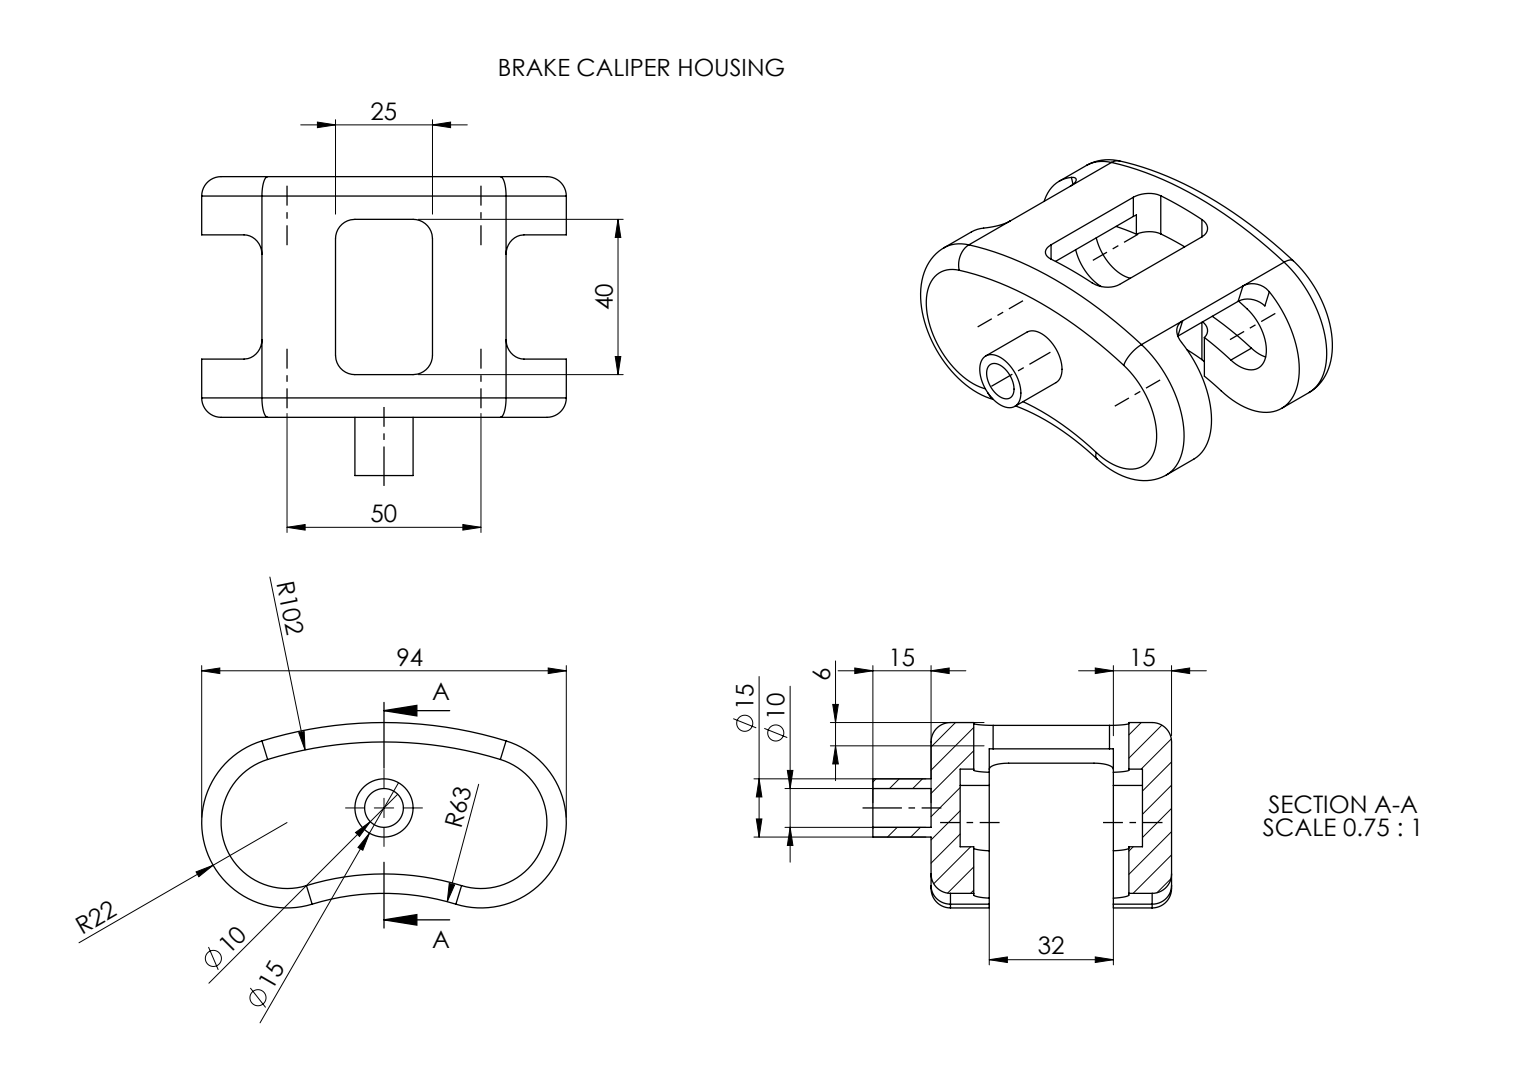
ISO-10303-21;
HEADER;
FILE_DESCRIPTION (('STEP AP214'),
    '1' );
FILE_NAME ('brake caliper housing.step',
    '2026-10-02T06:35:35',
    ( '' ),
    ( '' ),
    'SwSTEP 2.0',
    'SolidWorks 2026',
    '' );
FILE_SCHEMA (( 'AUTOMOTIVE_DESIGN' ));
ENDSEC;

DATA;
#2=DIRECTION ( 'NONE',  ( -1.000000000000000000, 0.000000000000000000, 0.000000000000000000 ) ) ;
#5=DIRECTION ( 'NONE',  ( -1.000000000000000000, 0.000000000000000000, 0.000000000000000000 ) ) ;
#22=AXIS2_PLACEMENT_3D ( 'NONE', #10002, #1881, #9007 ) ;
#27=VERTEX_POINT ( 'NONE', #8027 ) ;
#36=DIRECTION ( 'NONE',  ( -0.000000000000000000, -0.000000000000000000, -1.000000000000000000 ) ) ;
#37=CYLINDRICAL_SURFACE ( 'NONE', #355, 22.00000000000001421 ) ;
#47=CARTESIAN_POINT ( 'NONE',  ( 47.00000000000001421, 81.24038404635960831, -31.00000000000000000 ) ) ;
#48=FACE_BOUND ( 'NONE', #7708, .T. ) ;
#52=CARTESIAN_POINT ( 'NONE',  ( 36.08010649850015739, 100.2464683348682541, -16.00000000000000000 ) ) ;
#63=AXIS2_PLACEMENT_3D ( 'NONE', #8204, #12550, #5924 ) ;
#69=ADVANCED_FACE ( 'NONE', ( #14874 ), #12670, .F. ) ;
#73=EDGE_CURVE ( 'NONE', #4839, #9064, #14954, .T. ) ;
#82=CIRCLE ( 'NONE', #4216, 63.00000000000000000 ) ;
#86=LINE ( 'NONE', #9270, #8545 ) ;
#88=FACE_OUTER_BOUND ( 'NONE', #3167, .T. ) ;
#92=CARTESIAN_POINT ( 'NONE',  ( -10.00610186947451474, 106.5314655734664910, -19.33904518629106306 ) ) ;
#94=B_SPLINE_CURVE_WITH_KNOTS ( 'NONE', 3,
 ( #9442, #2468, #4910, #4826, #14091, #9801, #11106, #8665, #3618, #8738, #13380, #3696, #12955, #2552, #2981, #7235, #10661, #9522, #3776, #4761 ),
 .UNSPECIFIED., .F., .F.,
 ( 4, 2, 2, 2, 2, 2, 2, 2, 2, 4 ),
 ( 0.000000000000000000, 0.0009783709435495714819, 0.001467556415324351151, 0.001956741887099130821, 0.002935112830648695798, 0.003913483774198260774, 0.004891854717747825751, 0.005870225661297390728, 0.006848596604846954837, 0.007826967548396519814 ),
 .UNSPECIFIED. ) ;
#97=ORIENTED_EDGE ( 'NONE', *, *, #2089, .T. ) ;
#99=AXIS2_PLACEMENT_3D ( 'NONE', #4932, #13204, #7338 ) ;
#105=PLANE ( 'NONE',  #6564 ) ;
#111=DIRECTION ( 'NONE',  ( 1.000000000000000000, 0.000000000000000000, 0.000000000000000000 ) ) ;
#122=FACE_OUTER_BOUND ( 'NONE', #11782, .T. ) ;
#127=CARTESIAN_POINT ( 'NONE',  ( -10.20439220990035345, 94.45068983291282905, 19.21516791372541633 ) ) ;
#135=CARTESIAN_POINT ( 'NONE',  ( 12.50000000000000000, 40.62019202317980415, -16.00000000000000000 ) ) ;
#137=CARTESIAN_POINT ( 'NONE',  ( 10.21169758550232309, 62.16852661215632025, 19.23993411931846254 ) ) ;
#138=ORIENTED_EDGE ( 'NONE', *, *, #8514, .T. ) ;
#143=VERTEX_POINT ( 'NONE', #12163 ) ;
#155=ADVANCED_FACE ( 'NONE', ( #11017 ), #623, .F. ) ;
#179=CARTESIAN_POINT ( 'NONE',  ( 35.00000000000000000, 81.24038404635960831, 16.00000000000000000 ) ) ;
#200=DIRECTION ( 'NONE',  ( 0.000000000000000000, 0.000000000000000000, -1.000000000000000000 ) ) ;
#201=CARTESIAN_POINT ( 'NONE',  ( 11.10302805179279240, 62.01554028455485224, 18.51404809149990882 ) ) ;
#205=ORIENTED_EDGE ( 'NONE', *, *, #9389, .F. ) ;
#216=DIRECTION ( 'NONE',  ( 0.000000000000000000, 1.000000000000000000, 0.000000000000000000 ) ) ;
#220=ADVANCED_FACE ( 'NONE', ( #7246 ), #8324, .F. ) ;
#223=CARTESIAN_POINT ( 'NONE',  ( 25.00000000000000000, 81.24038404635960831, 26.00000000000000000 ) ) ;
#230=CARTESIAN_POINT ( 'NONE',  ( 12.39897948556635754, 61.76783392443436327, 16.00000000000000000 ) ) ;
#245=EDGE_LOOP ( 'NONE', ( #12911, #1425, #6697, #4365 ) ) ;
#253=FACE_OUTER_BOUND ( 'NONE', #11246, .T. ) ;
#257=AXIS2_PLACEMENT_3D ( 'NONE', #4931, #14259, #10909 ) ;
#259=VERTEX_POINT ( 'NONE', #10384 ) ;
#261=VECTOR ( 'NONE', #10408, 1000.000000000000000 ) ;
#266=EDGE_CURVE ( 'NONE', #4701, #13246, #688, .T. ) ;
#273=EDGE_CURVE ( 'NONE', #3532, #8404, #4570, .T. ) ;
#293=DIRECTION ( 'NONE',  ( 0.000000000000000000, 0.000000000000000000, -1.000000000000000000 ) ) ;
#296=CARTESIAN_POINT ( 'NONE',  ( 0.000000000000000000, 0.000000000000000000, 0.000000000000000000 ) ) ;
#298=FACE_OUTER_BOUND ( 'NONE', #14007, .T. ) ;
#304=AXIS2_PLACEMENT_3D ( 'NONE', #341, #1635, #4982 ) ;
#308=DIRECTION ( 'NONE',  ( 1.000000000000000000, 0.000000000000000000, 0.000000000000000000 ) ) ;
#310=CARTESIAN_POINT ( 'NONE',  ( 34.93100731845030538, 100.8740421756369585, -15.84356320956305986 ) ) ;
#315=AXIS2_PLACEMENT_3D ( 'NONE', #10797, #13156, #2521 ) ;
#320=ADVANCED_FACE ( 'NONE', ( #5891 ), #10531, .F. ) ;
#323=CARTESIAN_POINT ( 'NONE',  ( -9.716053034936795285, 106.5583837859906424, -19.49385781195229228 ) ) ;
#326=CARTESIAN_POINT ( 'NONE',  ( 31.47058823529413374, 102.2673069760056563, -31.00000000000000000 ) ) ;
#330=DIRECTION ( 'NONE',  ( 0.000000000000000000, 0.000000000000000000, -1.000000000000000000 ) ) ;
#331=VERTEX_POINT ( 'NONE', #8544 ) ;
#335=CARTESIAN_POINT ( 'NONE',  ( -33.08820577230232374, 101.7009610928537171, -14.78158739605038186 ) ) ;
#337=VERTEX_POINT ( 'NONE', #667 ) ;
#341=CARTESIAN_POINT ( 'NONE',  ( 25.00000000000000000, 81.24038404635960831, -31.00000000000000000 ) ) ;
#342=CIRCLE ( 'NONE', #8819, 75.00000000000001421 ) ;
#350=CARTESIAN_POINT ( 'NONE',  ( 10.43254889841015753, 62.13061131512487378, -19.05984907584257115 ) ) ;
#355=AXIS2_PLACEMENT_3D ( 'NONE', #4755, #11596, #10653 ) ;
#366=ORIENTED_EDGE ( 'NONE', *, *, #266, .F. ) ;
#369=AXIS2_PLACEMENT_3D ( 'NONE', #5329, #6524, #6684 ) ;
#370=ORIENTED_EDGE ( 'NONE', *, *, #5461, .F. ) ;
#373=DIRECTION ( 'NONE',  ( 0.000000000000000000, 0.000000000000000000, -1.000000000000000000 ) ) ;
#376=DIRECTION ( 'NONE',  ( 0.000000000000000000, 0.000000000000000000, 1.000000000000000000 ) ) ;
#377=DIRECTION ( 'NONE',  ( 1.000000000000000000, 0.000000000000000000, 0.000000000000000000 ) ) ;
#379=DIRECTION ( 'NONE',  ( -0.000000000000000000, -0.000000000000000000, -1.000000000000000000 ) ) ;
#382=EDGE_CURVE ( 'NONE', #697, #1597, #12234, .T. ) ;
#383=ORIENTED_EDGE ( 'NONE', *, *, #10951, .T. ) ;
#394=AXIS2_PLACEMENT_3D ( 'NONE', #10510, #36, #111 ) ;
#397=CARTESIAN_POINT ( 'NONE',  ( -11.83867104060235853, 106.3432143034623749, -17.50653253748098948 ) ) ;
#405=CARTESIAN_POINT ( 'NONE',  ( 12.46631608856921325, 100.2277185551817951, 15.67011936326128563 ) ) ;
#411=CARTESIAN_POINT ( 'NONE',  ( -31.71893208106490292, 102.1896529572239700, -12.62523369519216310 ) ) ;
#412=DIRECTION ( 'NONE',  ( 1.000000000000000000, 0.000000000000000000, 0.000000000000000000 ) ) ;
#428=CARTESIAN_POINT ( 'NONE',  ( -29.82779671029264890, 96.49509599019863515, -12.13403317654896973 ) ) ;
#450=CARTESIAN_POINT ( 'NONE',  ( -33.23060097332287199, 95.37689352056797532, 15.83317473434553690 ) ) ;
#453=LINE ( 'NONE', #9482, #11663 ) ;
#465=ORIENTED_EDGE ( 'NONE', *, *, #515, .F. ) ;
#467=B_SPLINE_CURVE_WITH_KNOTS ( 'NONE', 3,
 ( #4608, #10222, #15012, #14864, #7939, #12736, #1129, #12580, #13880, #3468, #13799, #2170, #3388, #6787, #11451, #12658, #1049, #8088 ),
 .UNSPECIFIED., .F., .F.,
 ( 4, 2, 2, 2, 2, 2, 2, 2, 4 ),
 ( 0.001002962753164633562, 0.001858089309406475969, 0.002713215865648318376, 0.003568342421890161216, 0.004423468978132004056, 0.005278595534373846029, 0.006133722090615688870, 0.006988848646857530843, 0.007843975203099373683 ),
 .UNSPECIFIED. ) ;
#470=CARTESIAN_POINT ( 'NONE',  ( 12.50000000000000000, 100.2235002382176248, 15.00000000000000000 ) ) ;
#478=DIRECTION ( 'NONE',  ( 0.000000000000000000, 0.000000000000000000, 1.000000000000000000 ) ) ;
#495=CARTESIAN_POINT ( 'NONE',  ( 11.45661564179884451, 61.94983405580222069, -18.07016506142804246 ) ) ;
#500=ORIENTED_EDGE ( 'NONE', *, *, #5316, .T. ) ;
#506=EDGE_CURVE ( 'NONE', #259, #13406, #11535, .T. ) ;
#508=VERTEX_POINT ( 'NONE', #11134 ) ;
#514=ORIENTED_EDGE ( 'NONE', *, *, #273, .T. ) ;
#515=EDGE_CURVE ( 'NONE', #15011, #5203, #11902, .T. ) ;
#527=EDGE_LOOP ( 'NONE', ( #759, #3459, #4325, #3794, #1827, #1753, #97, #3731 ) ) ;
#529=( GEOMETRIC_REPRESENTATION_CONTEXT ( 3 ) GLOBAL_UNCERTAINTY_ASSIGNED_CONTEXT ( ( #3045 ) ) GLOBAL_UNIT_ASSIGNED_CONTEXT ( ( #9128, #5633, #14911 ) ) REPRESENTATION_CONTEXT ( 'NONE', 'WORKASPACE' ) );
#530=EDGE_CURVE ( 'NONE', #7196, #1593, #12249, .T. ) ;
#531=CARTESIAN_POINT ( 'NONE',  ( 33.08545438203831424, 101.7020459634810976, -14.77901645503695605 ) ) ;
#532=EDGE_CURVE ( 'NONE', #4198, #5509, #6823, .T. ) ;
#564=LINE ( 'NONE', #14460, #13714 ) ;
#575=DIRECTION ( 'NONE',  ( 1.000000000000000000, 0.000000000000000000, 0.000000000000000000 ) ) ;
#576=PLANE ( 'NONE',  #9518 ) ;
#578=CARTESIAN_POINT ( 'NONE',  ( -30.00974697327757212, 96.43868009418278575, -12.76250177908513983 ) ) ;
#597=ADVANCED_FACE ( 'NONE', ( #8308 ), #37, .T. ) ;
#599=LINE ( 'NONE', #5072, #14330 ) ;
#609=ORIENTED_EDGE ( 'NONE', *, *, #9991, .T. ) ;
#613=CARTESIAN_POINT ( 'NONE',  ( -31.56843276583338209, 95.94012674102927463, 14.97885581718526105 ) ) ;
#623=CYLINDRICAL_SURFACE ( 'NONE', #7215, 4.999999999999998224 ) ;
#627=VECTOR ( 'NONE', #12367, 1000.000000000000000 ) ;
#629=CARTESIAN_POINT ( 'NONE',  ( 32.78625152019765210, 95.53054288192240051, -15.68243957109766207 ) ) ;
#638=AXIS2_PLACEMENT_3D ( 'NONE', #14300, #5118, #7308 ) ;
#641=CARTESIAN_POINT ( 'NONE',  ( -12.39897948556635754, 94.18739463280904545, 16.00000000000000000 ) ) ;
#643=EDGE_LOOP ( 'NONE', ( #12832, #6192, #9404, #8598 ) ) ;
#646=CARTESIAN_POINT ( 'NONE',  ( 25.00000000000000000, 81.24038404635960831, 31.00000000000000000 ) ) ;
#650=ORIENTED_EDGE ( 'NONE', *, *, #11602, .F. ) ;
#658=CARTESIAN_POINT ( 'NONE',  ( 8.076099607191862262, 62.48290387921808531, -20.00000000000000355 ) ) ;
#659=CARTESIAN_POINT ( 'NONE',  ( 30.00000000000000355, 97.48846085563152997, 31.00000000000000000 ) ) ;
#666=CARTESIAN_POINT ( 'NONE',  ( -7.499999999999996447, 85.00000000000000000, 31.00000000000000000 ) ) ;
#667=CARTESIAN_POINT ( 'NONE',  ( 29.70588235294119173, 96.53269163155674448, 10.99999999999999645 ) ) ;
#672=CARTESIAN_POINT ( 'NONE',  ( -12.46631608856921325, 100.2277185551817951, -15.67011936326128563 ) ) ;
#673=CARTESIAN_POINT ( 'NONE',  ( -19.99999999999998934, 64.99230723708770086, 31.00000000000000000 ) ) ;
#674=APPLICATION_CONTEXT ( 'automotive_design' ) ;
#675=( LENGTH_UNIT ( ) NAMED_UNIT ( * ) SI_UNIT ( .MILLI., .METRE. ) );
#681=AXIS2_PLACEMENT_3D ( 'NONE', #14508, #12588, #11545 ) ;
#684=CARTESIAN_POINT ( 'NONE',  ( -33.83210567914650113, 95.16559600367024530, 15.96768719852781615 ) ) ;
#686=EDGE_CURVE ( 'NONE', #1445, #27, #6861, .T. ) ;
#687=DIRECTION ( 'NONE',  ( -0.000000000000000000, -0.000000000000000000, -1.000000000000000000 ) ) ;
#688=CIRCLE ( 'NONE', #3352, 75.00000000000001421 ) ;
#697=VERTEX_POINT ( 'NONE', #5872 ) ;
#698=CARTESIAN_POINT ( 'NONE',  ( 0.000000000000000000, 0.000000000000000000, 31.00000000000000000 ) ) ;
#699=EDGE_CURVE ( 'NONE', #5509, #721, #10511, .T. ) ;
#705=CARTESIAN_POINT ( 'NONE',  ( -11.47921512510733422, 94.30438942219511489, -18.08174836683881992 ) ) ;
#714=DIRECTION ( 'NONE',  ( 0.000000000000000000, 0.000000000000000000, 1.000000000000000000 ) ) ;
#717=DIRECTION ( 'NONE',  ( -0.000000000000000000, -0.000000000000000000, 1.000000000000000000 ) ) ;
#720=ADVANCED_FACE ( 'NONE', ( #6388 ), #10963, .T. ) ;
#721=VERTEX_POINT ( 'NONE', #13248 ) ;
#725=CARTESIAN_POINT ( 'NONE',  ( 11.83526203526748333, 106.3435961965382290, -17.51264358390114140 ) ) ;
#730=ORIENTED_EDGE ( 'NONE', *, *, #3331, .F. ) ;
#736=CARTESIAN_POINT ( 'NONE',  ( 35.50766591049263354, 100.5715065882092460, 15.96896126722778497 ) ) ;
#739=EDGE_LOOP ( 'NONE', ( #11744, #3948, #14361, #10298 ) ) ;
#754=CARTESIAN_POINT ( 'NONE',  ( -31.63177518854774206, 102.2170822241992454, 12.29884221335728789 ) ) ;
#755=ORIENTED_EDGE ( 'NONE', *, *, #10454, .F. ) ;
#759=ORIENTED_EDGE ( 'NONE', *, *, #10762, .F. ) ;
#761=ORIENTED_EDGE ( 'NONE', *, *, #6262, .F. ) ;
#762=CARTESIAN_POINT ( 'NONE',  ( -34.44830544488820578, 94.94374256356071839, 16.00000000000000000 ) ) ;
#777=CARTESIAN_POINT ( 'NONE',  ( 29.86020745210524296, 96.48508785265609333, -12.30285360678859696 ) ) ;
#778=DIRECTION ( 'NONE',  ( -0.000000000000000000, -0.000000000000000000, -1.000000000000000000 ) ) ;
#798=DIRECTION ( 'NONE',  ( 1.000000000000000000, 0.000000000000000000, 0.000000000000000000 ) ) ;
#801=AXIS2_PLACEMENT_3D ( 'NONE', #7638, #12285, #12205 ) ;
#803=LINE ( 'NONE', #5569, #8515 ) ;
#804=ORIENTED_EDGE ( 'NONE', *, *, #9181, .F. ) ;
#806=DIRECTION ( 'NONE',  ( -1.000000000000000000, 0.000000000000000000, -0.000000000000000000 ) ) ;
#815=CARTESIAN_POINT ( 'NONE',  ( 11.47921512510733422, 94.30438942219511489, 18.08174836683881992 ) ) ;
#818=CARTESIAN_POINT ( 'NONE',  ( 29.70588235294119173, 96.53269163155674448, -79.80561291909842225 ) ) ;
#819=ORIENTED_EDGE ( 'NONE', *, *, #273, .F. ) ;
#820=VECTOR ( 'NONE', #3846, 1000.000000000000000 ) ;
#822=EDGE_LOOP ( 'NONE', ( #2151, #1128, #4387, #7220 ) ) ;
#827=ORIENTED_EDGE ( 'NONE', *, *, #1988, .F. ) ;
#831=CARTESIAN_POINT ( 'NONE',  ( -34.93100731845028406, 100.8740421756369301, 15.84356320956306341 ) ) ;
#833=CARTESIAN_POINT ( 'NONE',  ( -30.00000000000000711, 97.48846085563154418, -26.00000000000000000 ) ) ;
#835=ADVANCED_FACE ( 'NONE', ( #5120 ), #6173, .T. ) ;
#842=AXIS2_PLACEMENT_3D ( 'NONE', #10115, #4783, #2574 ) ;
#844=EDGE_CURVE ( 'NONE', #2618, #331, #564, .T. ) ;
#845=DIRECTION ( 'NONE',  ( 0.9557692240748192347, 0.2941176470588224845, 0.000000000000000000 ) ) ;
#854=CARTESIAN_POINT ( 'NONE',  ( 8.076072847916476505, 62.48290708766281654, 19.99999999999999645 ) ) ;
#857=CARTESIAN_POINT ( 'NONE',  ( 31.56843276583338920, 95.94012674102923199, -14.97885581718525572 ) ) ;
#858=CIRCLE ( 'NONE', #6169, 101.0000000000000284 ) ;
#863=AXIS2_PLACEMENT_3D ( 'NONE', #3956, #5244, #8715 ) ;
#865=CARTESIAN_POINT ( 'NONE',  ( -7.500000000000000000, 94.70348462437907244, -20.00000000000000000 ) ) ;
#868=ORIENTED_EDGE ( 'NONE', *, *, #10994, .T. ) ;
#878=CARTESIAN_POINT ( 'NONE',  ( 25.00000000000000000, 81.24038404635960831, -31.00000000000000000 ) ) ;
#882=CARTESIAN_POINT ( 'NONE',  ( 17.27884612037405887, 39.14960378788569528, -16.00000000000000000 ) ) ;
#885=DIRECTION ( 'NONE',  ( -1.000000000000000000, 0.000000000000000000, 0.000000000000000000 ) ) ;
#888=CARTESIAN_POINT ( 'NONE',  ( 12.24154204929785372, 106.2975094407664471, -16.61985167119453877 ) ) ;
#897=CARTESIAN_POINT ( 'NONE',  ( 12.07539369549097863, 94.22990561005788379, 17.09692597381455315 ) ) ;
#902=EDGE_CURVE ( 'NONE', #13406, #12353, #9331, .T. ) ;
#910=PLANE ( 'NONE',  #6070 ) ;
#911=CARTESIAN_POINT ( 'NONE',  ( -35.50612649840985569, 100.5723974928649085, 15.96895346309148245 ) ) ;
#921=EDGE_CURVE ( 'NONE', #4010, #3168, #2065, .T. ) ;
#933=CARTESIAN_POINT ( 'NONE',  ( 30.88253268887308423, 96.16299873708393875, 14.30432816676292163 ) ) ;
#942=FACE_OUTER_BOUND ( 'NONE', #13951, .T. ) ;
#944=VERTEX_POINT ( 'NONE', #2076 ) ;
#950=DIRECTION ( 'NONE',  ( 0.000000000000000000, 0.000000000000000000, -1.000000000000000000 ) ) ;
#960=ADVANCED_FACE ( 'NONE', ( #11195 ), #9886, .T. ) ;
#962=CARTESIAN_POINT ( 'NONE',  ( 12.28362713749409529, 94.20257980066446635, 16.56510878681792320 ) ) ;
#970=CARTESIAN_POINT ( 'NONE',  ( -36.08010649850015028, 100.2464683348682541, -16.00000000000000000 ) ) ;
#978=EDGE_CURVE ( 'NONE', #7811, #2618, #11566, .T. ) ;
#979=EDGE_CURVE ( 'NONE', #4839, #10382, #4953, .T. ) ;
#988=COLOUR_RGB ( '', 0.31764706, 0.68627451, 0.89019608) ;
#994=CIRCLE ( 'NONE', #7761, 10.00000000000000355 ) ;
#1015=DIRECTION ( 'NONE',  ( -0.9557692240748186796, -0.2941176470588241498, 0.000000000000000000 ) ) ;
#1025=ORIENTED_EDGE ( 'NONE', *, *, #14569, .T. ) ;
#1030=EDGE_LOOP ( 'NONE', ( #7241, #8999, #5615, #1735 ) ) ;
#1035=CARTESIAN_POINT ( 'NONE',  ( 7.830013896347493230, 106.7136370351866077, -20.00000000000000355 ) ) ;
#1040=ORIENTED_EDGE ( 'NONE', *, *, #14569, .F. ) ;
#1041=ORIENTED_EDGE ( 'NONE', *, *, #6655, .T. ) ;
#1042=CARTESIAN_POINT ( 'NONE',  ( -11.10302805179279240, 62.01554028455485224, -18.51404809149991237 ) ) ;
#1049=CARTESIAN_POINT ( 'NONE',  ( 7.787661217455939422, 74.59514674284385194, 20.00000000000000000 ) ) ;
#1052=LINE ( 'NONE', #5668, #11439 ) ;
#1057=VECTOR ( 'NONE', #14220, 1000.000000000000114 ) ;
#1079=VECTOR ( 'NONE', #8441, 1000.000000000000000 ) ;
#1086=ORIENTED_EDGE ( 'NONE', *, *, #7949, .F. ) ;
#1087=DIRECTION ( 'NONE',  ( -1.000000000000000000, -6.217248937900876626E-15, 0.000000000000000000 ) ) ;
#1091=CARTESIAN_POINT ( 'NONE',  ( -12.33783400350010595, 106.2863213744706172, 16.30550365830425363 ) ) ;
#1092=DIRECTION ( 'NONE',  ( 1.000000000000000000, 0.000000000000000000, 0.000000000000000000 ) ) ;
#1099=CARTESIAN_POINT ( 'NONE',  ( 7.500000000000000888, 106.2673515243510991, -20.00000000000000000 ) ) ;
#1118=ORIENTED_EDGE ( 'NONE', *, *, #13189, .T. ) ;
#1125=EDGE_CURVE ( 'NONE', #13289, #1809, #11865, .T. ) ;
#1128=ORIENTED_EDGE ( 'NONE', *, *, #13331, .F. ) ;
#1129=CARTESIAN_POINT ( 'NONE',  ( 11.45967689402250755, 74.11957758926655515, 18.06636219913714214 ) ) ;
#1137=ORIENTED_EDGE ( 'NONE', *, *, #10454, .T. ) ;
#1158=VERTEX_POINT ( 'NONE', #8439 ) ;
#1159=DIRECTION ( 'NONE',  ( -1.000000000000000000, 0.000000000000000000, 0.000000000000000000 ) ) ;
#1162=DIRECTION ( 'NONE',  ( 0.000000000000000000, -1.000000000000000000, 0.000000000000000000 ) ) ;
#1166=ORIENTED_EDGE ( 'NONE', *, *, #6232, .T. ) ;
#1172=DIRECTION ( 'NONE',  ( 1.000000000000000000, 0.000000000000000000, 0.000000000000000000 ) ) ;
#1176=DIRECTION ( 'NONE',  ( 1.000000000000000000, 0.000000000000000000, 0.000000000000000000 ) ) ;
#1182=CARTESIAN_POINT ( 'NONE',  ( -27.94117647058823550, 90.79807628710781842, 13.50000000000000533 ) ) ;
#1197=EDGE_LOOP ( 'NONE', ( #4372, #1544, #6897, #8188 ) ) ;
#1203=ADVANCED_FACE ( 'NONE', ( #1394 ), #3893, .F. ) ;
#1209=AXIS2_PLACEMENT_3D ( 'NONE', #2497, #13132, #377 ) ;
#1219=ORIENTED_EDGE ( 'NONE', *, *, #11069, .T. ) ;
#1220=DIRECTION ( 'NONE',  ( -0.000000000000000000, -0.000000000000000000, -1.000000000000000000 ) ) ;
#1225=CYLINDRICAL_SURFACE ( 'NONE', #2799, 75.00000000000001421 ) ;
#1226=CARTESIAN_POINT ( 'NONE',  ( -9.104688129943026453, 106.6120509519916766, 19.73833377876426809 ) ) ;
#1227=CARTESIAN_POINT ( 'NONE',  ( -25.00000000000000000, 81.24038404635962252, 13.50000000000000533 ) ) ;
#1231=CIRCLE ( 'NONE', #1719, 95.00000000000001421 ) ;
#1276=ORIENTED_EDGE ( 'NONE', *, *, #13026, .T. ) ;
#1290=EDGE_LOOP ( 'NONE', ( #7125, #7121, #500, #6084, #514, #11735, #1897, #13046 ) ) ;
#1292=DIRECTION ( 'NONE',  ( 0.2941176470588243164, 0.9557692240748186796, 0.000000000000000000 ) ) ;
#1294=EDGE_CURVE ( 'NONE', #4446, #1777, #1831, .T. ) ;
#1302=DIRECTION ( 'NONE',  ( 0.000000000000000000, 0.000000000000000000, -1.000000000000000000 ) ) ;
#1305=CARTESIAN_POINT ( 'NONE',  ( -8.791121401460923579, 106.6383652286473023, 19.83320147728688454 ) ) ;
#1307=DIRECTION ( 'NONE',  ( -1.000000000000000000, 0.000000000000000000, 0.000000000000000000 ) ) ;
#1316=DIRECTION ( 'NONE',  ( -0.000000000000000000, -0.000000000000000000, 1.000000000000000000 ) ) ;
#1334=DIRECTION ( 'NONE',  ( 0.000000000000000000, 1.000000000000000000, 0.000000000000000000 ) ) ;
#1341=CIRCLE ( 'NONE', #4739, 10.00000000000000178 ) ;
#1361=ORIENTED_EDGE ( 'NONE', *, *, #9655, .T. ) ;
#1362=CARTESIAN_POINT ( 'NONE',  ( 12.39897948556635754, 73.96800191783272282, -16.00000000000000000 ) ) ;
#1371=EDGE_LOOP ( 'NONE', ( #10075, #6028, #9501, #13452, #10870, #9766, #4151, #3921 ) ) ;
#1388=CARTESIAN_POINT ( 'NONE',  ( 12.39897948556635754, 94.18739463280904545, -16.00000000000000000 ) ) ;
#1392=VERTEX_POINT ( 'NONE', #12609 ) ;
#1394=FACE_OUTER_BOUND ( 'NONE', #1945, .T. ) ;
#1397=LINE ( 'NONE', #326, #1079 ) ;
#1421=ORIENTED_EDGE ( 'NONE', *, *, #8740, .F. ) ;
#1423=DIRECTION ( 'NONE',  ( 0.000000000000000000, 0.000000000000000000, -1.000000000000000000 ) ) ;
#1425=ORIENTED_EDGE ( 'NONE', *, *, #8652, .F. ) ;
#1426=ORIENTED_EDGE ( 'NONE', *, *, #4047, .T. ) ;
#1428=ORIENTED_EDGE ( 'NONE', *, *, #9477, .F. ) ;
#1429=DIRECTION ( 'NONE',  ( -1.000000000000000000, 0.000000000000000000, 0.000000000000000000 ) ) ;
#1430=CARTESIAN_POINT ( 'NONE',  ( -10.21287289150292921, 74.30275811153845211, 19.23918552186208686 ) ) ;
#1437=CYLINDRICAL_SURFACE ( 'NONE', #6308, 5.000000000000000888 ) ;
#1438=FACE_OUTER_BOUND ( 'NONE', #9792, .T. ) ;
#1445=VERTEX_POINT ( 'NONE', #5618 ) ;
#1447=CARTESIAN_POINT ( 'NONE',  ( 31.72333741318945144, 102.1879147510518777, -12.61437971294004434 ) ) ;
#1448=DIRECTION ( 'NONE',  ( 0.000000000000000000, 0.000000000000000000, 1.000000000000000000 ) ) ;
#1466=PLANE ( 'NONE',  #7745 ) ;
#1482=CARTESIAN_POINT ( 'NONE',  ( -22.05882352941176450, 71.68269180561142662, -16.00000000000000000 ) ) ;
#1495=VERTEX_POINT ( 'NONE', #2031 ) ;
#1506=DIRECTION ( 'NONE',  ( 0.000000000000000000, 0.000000000000000000, -1.000000000000000000 ) ) ;
#1508=CYLINDRICAL_SURFACE ( 'NONE', #257, 5.000000000000000888 ) ;
#1513=DIRECTION ( 'NONE',  ( 1.000000000000000000, 0.000000000000000000, 0.000000000000000000 ) ) ;
#1527=CARTESIAN_POINT ( 'NONE',  ( 0.000000000000000000, 0.000000000000000000, 31.00000000000000000 ) ) ;
#1533=DIRECTION ( 'NONE',  ( 1.000000000000000000, 0.000000000000000000, 0.000000000000000000 ) ) ;
#1535=EDGE_CURVE ( 'NONE', #6344, #3532, #3101, .T. ) ;
#1542=VERTEX_POINT ( 'NONE', #10080 ) ;
#1543=CIRCLE ( 'NONE', #14391, 5.000000000000001776 ) ;
#1544=ORIENTED_EDGE ( 'NONE', *, *, #2587, .F. ) ;
#1553=CARTESIAN_POINT ( 'NONE',  ( 18.52941176470587692, 60.21346111671358159, -31.00000000000000000 ) ) ;
#1576=B_SPLINE_CURVE_WITH_KNOTS ( 'NONE', 3,
 ( #10284, #1035, #14772, #13625, #6770, #11436, #6705, #5507, #8912, #11205, #13547, #4373, #3155, #725, #8987, #888, #12498, #4304, #2091, #11355 ),
 .UNSPECIFIED., .F., .F.,
 ( 4, 2, 2, 2, 2, 2, 2, 2, 2, 4 ),
 ( 0.000000000000000000, 0.0009783702772842371286, 0.001467555415926354934, 0.001956740554568472523, 0.002935110831852707266, 0.003913481109136941576, 0.004891851386421175452, 0.005870221663705411062, 0.006848591940989644938, 0.007826962218273879682 ),
 .UNSPECIFIED. ) ;
#1586=DIRECTION ( 'NONE',  ( 0.000000000000000000, 0.000000000000000000, -1.000000000000000000 ) ) ;
#1588=CARTESIAN_POINT ( 'NONE',  ( 36.08010649850015739, 100.2464683348682541, 16.00000000000000000 ) ) ;
#1593=VERTEX_POINT ( 'NONE', #12439 ) ;
#1594=CARTESIAN_POINT ( 'NONE',  ( 0.000000000000000000, 0.000000000000000000, 25.99999999999999645 ) ) ;
#1595=AXIS2_PLACEMENT_3D ( 'NONE', #9325, #5829, #9393 ) ;
#1597=VERTEX_POINT ( 'NONE', #12294 ) ;
#1617=PLANE ( 'NONE',  #315 ) ;
#1618=EDGE_LOOP ( 'NONE', ( #11219, #4942, #12564, #4968 ) ) ;
#1625=CARTESIAN_POINT ( 'NONE',  ( -15.11621636258860590, 32.12188890498260463, 16.00000000000000000 ) ) ;
#1635=DIRECTION ( 'NONE',  ( -0.000000000000000000, -0.000000000000000000, 1.000000000000000000 ) ) ;
#1637=ORIENTED_EDGE ( 'NONE', *, *, #7630, .F. ) ;
#1638=LINE ( 'NONE', #7392, #11678 ) ;
#1642=CARTESIAN_POINT ( 'NONE',  ( -12.50000000000000000, 100.2235002382176248, -79.80561291909842225 ) ) ;
#1644=ORIENTED_EDGE ( 'NONE', *, *, #10929, .T. ) ;
#1645=ORIENTED_EDGE ( 'NONE', *, *, #4912, .T. ) ;
#1647=DIRECTION ( 'NONE',  ( 0.000000000000000000, 0.000000000000000000, -1.000000000000000000 ) ) ;
#1651=ORIENTED_EDGE ( 'NONE', *, *, #699, .T. ) ;
#1654=DIRECTION ( 'NONE',  ( -0.000000000000000000, -0.000000000000000000, 1.000000000000000000 ) ) ;
#1659=ORIENTED_EDGE ( 'NONE', *, *, #978, .T. ) ;
#1670=CARTESIAN_POINT ( 'NONE',  ( 31.47058823529413374, 102.2673069760056563, -10.99999999999999645 ) ) ;
#1678=DIRECTION ( 'NONE',  ( -0.000000000000000000, -0.000000000000000000, 1.000000000000000000 ) ) ;
#1679=ORIENTED_EDGE ( 'NONE', *, *, #8420, .F. ) ;
#1681=AXIS2_PLACEMENT_3D ( 'NONE', #5773, #4732, #11792 ) ;
#1684=CARTESIAN_POINT ( 'NONE',  ( 25.00000000000000000, 81.24038404635960831, 16.00000000000000000 ) ) ;
#1689=VERTEX_POINT ( 'NONE', #5958 ) ;
#1693=CARTESIAN_POINT ( 'NONE',  ( -34.51370081393726963, 101.0775402828204506, -15.68973407569667167 ) ) ;
#1702=EDGE_CURVE ( 'NONE', #14939, #14649, #3395, .T. ) ;
#1711=DIRECTION ( 'NONE',  ( -0.000000000000000000, -0.000000000000000000, -1.000000000000000000 ) ) ;
#1719=AXIS2_PLACEMENT_3D ( 'NONE', #9468, #11843, #14040 ) ;
#1720=CARTESIAN_POINT ( 'NONE',  ( 7.500000000000000000, 59.24038404635959409, 15.00000000000000000 ) ) ;
#1722=CARTESIAN_POINT ( 'NONE',  ( 12.39897948556635754, 100.2360479454198696, -16.00000000000000000 ) ) ;
#1735=ORIENTED_EDGE ( 'NONE', *, *, #2918, .T. ) ;
#1740=CYLINDRICAL_SURFACE ( 'NONE', #12850, 5.000000000000000888 ) ;
#1753=ORIENTED_EDGE ( 'NONE', *, *, #2736, .F. ) ;
#1762=DIRECTION ( 'NONE',  ( 1.000000000000000000, 0.000000000000000000, 0.000000000000000000 ) ) ;
#1764=ORIENTED_EDGE ( 'NONE', *, *, #4407, .F. ) ;
#1765=DIRECTION ( 'NONE',  ( -1.000000000000000000, 0.000000000000000000, -0.000000000000000000 ) ) ;
#1777=VERTEX_POINT ( 'NONE', #4916 ) ;
#1780=DIRECTION ( 'NONE',  ( 0.000000000000000000, 0.000000000000000000, 1.000000000000000000 ) ) ;
#1782=AXIS2_PLACEMENT_3D ( 'NONE', #2564, #2859, #7475 ) ;
#1784=ORIENTED_EDGE ( 'NONE', *, *, #6798, .T. ) ;
#1791=VECTOR ( 'NONE', #11295, 1000.000000000000000 ) ;
#1792=DIRECTION ( 'NONE',  ( 0.000000000000000000, 0.000000000000000000, -1.000000000000000000 ) ) ;
#1797=EDGE_CURVE ( 'NONE', #14203, #697, #9116, .T. ) ;
#1799=DIRECTION ( 'NONE',  ( -1.000000000000000000, 0.000000000000000000, 0.000000000000000000 ) ) ;
#1800=ADVANCED_FACE ( 'NONE', ( #7469 ), #3848, .T. ) ;
#1803=ORIENTED_EDGE ( 'NONE', *, *, #10490, .F. ) ;
#1808=FACE_OUTER_BOUND ( 'NONE', #7199, .T. ) ;
#1809=VERTEX_POINT ( 'NONE', #10976 ) ;
#1811=DIRECTION ( 'NONE',  ( 1.000000000000000000, -1.953992523340275511E-14, 0.000000000000000000 ) ) ;
#1820=CARTESIAN_POINT ( 'NONE',  ( -32.08430773043616568, 95.76884182151509606, 15.34120815717650110 ) ) ;
#1827=ORIENTED_EDGE ( 'NONE', *, *, #7210, .T. ) ;
#1831=LINE ( 'NONE', #3276, #6297 ) ;
#1833=AXIS2_PLACEMENT_3D ( 'NONE', #7575, #4260, #7722 ) ;
#1843=DIRECTION ( 'NONE',  ( 0.000000000000000000, 0.000000000000000000, 1.000000000000000000 ) ) ;
#1849=CARTESIAN_POINT ( 'NONE',  ( 18.52941176470587692, 60.21346111671358159, -16.00000000000000000 ) ) ;
#1852=CARTESIAN_POINT ( 'NONE',  ( 12.34206246762915882, 94.19488728021195811, -16.27883530325393835 ) ) ;
#1854=EDGE_CURVE ( 'NONE', #14085, #4528, #14168, .T. ) ;
#1856=CIRCLE ( 'NONE', #7184, 22.00000000000001421 ) ;
#1858=ORIENTED_EDGE ( 'NONE', *, *, #8427, .T. ) ;
#1866=ORIENTED_EDGE ( 'NONE', *, *, #11969, .F. ) ;
#1868=ORIENTED_EDGE ( 'NONE', *, *, #13043, .F. ) ;
#1870=DIRECTION ( 'NONE',  ( -1.000000000000000000, -4.440892098500626162E-15, 0.000000000000000000 ) ) ;
#1876=CARTESIAN_POINT ( 'NONE',  ( -12.39897948556635754, 100.2360479454198696, -16.00000000000000000 ) ) ;
#1881=DIRECTION ( 'NONE',  ( -0.000000000000000000, -0.000000000000000000, -1.000000000000000000 ) ) ;
#1897=ORIENTED_EDGE ( 'NONE', *, *, #4427, .F. ) ;
#1899=DIRECTION ( 'NONE',  ( 1.000000000000000000, -3.552713678800500929E-15, 0.000000000000000000 ) ) ;
#1905=CARTESIAN_POINT ( 'NONE',  ( 47.00000000000001421, 81.24038404635960831, 16.00000000000000000 ) ) ;
#1916=ORIENTED_EDGE ( 'NONE', *, *, #11920, .F. ) ;
#1920=VERTEX_POINT ( 'NONE', #666 ) ;
#1928=EDGE_CURVE ( 'NONE', #4839, #11834, #12993, .T. ) ;
#1937=AXIS2_PLACEMENT_3D ( 'NONE', #14153, #9363, #9287 ) ;
#1938=CYLINDRICAL_SURFACE ( 'NONE', #8862, 5.000000000000000888 ) ;
#1941=CIRCLE ( 'NONE', #5811, 63.00000000000000000 ) ;
#1945=EDGE_LOOP ( 'NONE', ( #2514, #8632, #7779, #11237 ) ) ;
#1958=CARTESIAN_POINT ( 'NONE',  ( -12.39897948556635754, 61.76783392443436327, -16.00000000000000000 ) ) ;
#1968=VECTOR ( 'NONE', #6575, 1000.000000000000000 ) ;
#1976=ADVANCED_FACE ( 'NONE', ( #14550 ), #14777, .F. ) ;
#1982=DIRECTION ( 'NONE',  ( 0.000000000000000000, 0.000000000000000000, -1.000000000000000000 ) ) ;
#1988=EDGE_CURVE ( 'NONE', #8172, #5421, #5442, .T. ) ;
#2000=CARTESIAN_POINT ( 'NONE',  ( 11.63111172283970518, 94.28541358805125583, -17.83102282485378254 ) ) ;
#2002=DIRECTION ( 'NONE',  ( -1.000000000000000000, 0.000000000000000000, 0.000000000000000000 ) ) ;
#2003=CIRCLE ( 'NONE', #14123, 63.00000000000000000 ) ;
#2016=CARTESIAN_POINT ( 'NONE',  ( -7.500000000000000888, 59.24038404635959409, 15.00000000000000000 ) ) ;
#2017=CARTESIAN_POINT ( 'NONE',  ( 0.000000000000000000, 0.000000000000000000, -26.00000000000000000 ) ) ;
#2018=AXIS2_PLACEMENT_3D ( 'NONE', #5999, #4885, #14142 ) ;
#2019=DIRECTION ( 'NONE',  ( -0.9557692240748186796, 0.2941176470588241498, -1.531423350357148967E-16 ) ) ;
#2031=CARTESIAN_POINT ( 'NONE',  ( 34.44830544488820578, 94.94374256356071839, -16.00000000000000000 ) ) ;
#2032=ADVANCED_FACE ( 'NONE', ( #12122 ), #1938, .F. ) ;
#2036=CARTESIAN_POINT ( 'NONE',  ( -31.59365702568382872, 102.2290646705776140, 12.13969626787233480 ) ) ;
#2039=EDGE_LOOP ( 'NONE', ( #6393, #1428, #10649, #1916 ) ) ;
#2042=CARTESIAN_POINT ( 'NONE',  ( -7.500000000000000000, 94.70348462437907244, -20.00000000000000000 ) ) ;
#2053=VECTOR ( 'NONE', #14016, 1000.000000000000000 ) ;
#2056=CARTESIAN_POINT ( 'NONE',  ( 9.717538815323484513, 62.24844358264333266, 19.51802576651051879 ) ) ;
#2062=CARTESIAN_POINT ( 'NONE',  ( 0.000000000000000000, 0.000000000000000000, -23.50000000000000000 ) ) ;
#2065=CIRCLE ( 'NONE', #2767, 95.00000000000001421 ) ;
#2072=CARTESIAN_POINT ( 'NONE',  ( -29.70588235294118107, 96.53269163155674448, 10.99999999999999645 ) ) ;
#2073=AXIS2_PLACEMENT_3D ( 'NONE', #14423, #4027, #8641 ) ;
#2076=CARTESIAN_POINT ( 'NONE',  ( 12.39897948556635754, 100.2360479454198696, -16.00000000000000000 ) ) ;
#2089=EDGE_CURVE ( 'NONE', #11234, #5062, #7461, .T. ) ;
#2091=CARTESIAN_POINT ( 'NONE',  ( 12.50000000000000178, 106.2673515243511275, -15.33085973118640055 ) ) ;
#2097=CARTESIAN_POINT ( 'NONE',  ( -10.21169758550232309, 62.16852661215632025, -19.23993411931846609 ) ) ;
#2098=CARTESIAN_POINT ( 'NONE',  ( 32.65306121041741960, 101.8676703390407283, 14.32076206672372365 ) ) ;
#2104=DIRECTION ( 'NONE',  ( 0.000000000000000000, 0.000000000000000000, -1.000000000000000000 ) ) ;
#2108=ORIENTED_EDGE ( 'NONE', *, *, #2903, .F. ) ;
#2115=EDGE_LOOP ( 'NONE', ( #13214, #3973, #6177, #9245 ) ) ;
#2124=EDGE_CURVE ( 'NONE', #8389, #4446, #14462, .T. ) ;
#2129=DIRECTION ( 'NONE',  ( -0.000000000000000000, -0.000000000000000000, 1.000000000000000000 ) ) ;
#2138=CARTESIAN_POINT ( 'NONE',  ( -12.46747951117848885, 106.2711918341631900, 15.65812229356676433 ) ) ;
#2145=CARTESIAN_POINT ( 'NONE',  ( 25.00000000000000000, 81.24038404635960831, -26.00000000000000000 ) ) ;
#2151=ORIENTED_EDGE ( 'NONE', *, *, #10847, .F. ) ;
#2160=CARTESIAN_POINT ( 'NONE',  ( -8.635061085254617907, 62.40781208424768778, -19.90323072647615987 ) ) ;
#2161=CARTESIAN_POINT ( 'NONE',  ( 7.500000000000000000, 94.70348462437907244, 20.00000000000000000 ) ) ;
#2165=EDGE_CURVE ( 'NONE', #697, #11955, #4599, .T. ) ;
#2170=CARTESIAN_POINT ( 'NONE',  ( 9.706343076449424956, 74.36968214894433515, 19.49591231693629112 ) ) ;
#2180=CARTESIAN_POINT ( 'NONE',  ( 12.50000000000000000, 100.2235002382176248, -79.80561291909842225 ) ) ;
#2182=EDGE_CURVE ( 'NONE', #10943, #3127, #9122, .T. ) ;
#2184=PRODUCT_DEFINITION_FORMATION_WITH_SPECIFIED_SOURCE ( 'ANY', '', #11452, .NOT_KNOWN. ) ;
#2192=DIRECTION ( 'NONE',  ( 0.000000000000000000, -1.000000000000000000, 0.000000000000000000 ) ) ;
#2197=AXIS2_PLACEMENT_3D ( 'NONE', #6730, #12898, #10320 ) ;
#2198=CARTESIAN_POINT ( 'NONE',  ( -25.00000000000000000, 81.24038404635962252, -16.00000000000000000 ) ) ;
#2222=CARTESIAN_POINT ( 'NONE',  ( 0.000000000000000000, 0.000000000000000000, 13.50000000000000533 ) ) ;
#2235=CARTESIAN_POINT ( 'NONE',  ( -12.50000000000000000, 106.2673515243510991, -31.00000000000000000 ) ) ;
#2244=EDGE_LOOP ( 'NONE', ( #9568, #3382, #5426, #11140 ) ) ;
#2245=ORIENTED_EDGE ( 'NONE', *, *, #10151, .F. ) ;
#2259=DIRECTION ( 'NONE',  ( 0.000000000000000000, -1.000000000000000000, 0.000000000000000000 ) ) ;
#2261=ORIENTED_EDGE ( 'NONE', *, *, #8888, .T. ) ;
#2264=VERTEX_POINT ( 'NONE', #14079 ) ;
#2272=EDGE_CURVE ( 'NONE', #10943, #8733, #2540, .T. ) ;
#2275=FACE_OUTER_BOUND ( 'NONE', #2244, .T. ) ;
#2277=CARTESIAN_POINT ( 'NONE',  ( -36.08010649850015028, 100.2464683348682684, 16.00000000000000000 ) ) ;
#2279=B_SPLINE_CURVE_WITH_KNOTS ( 'NONE', 3,
 ( #4722, #3351, #3280, #13835, #13988, #6974, #3582, #3508, #8200, #8129, #933, #11631, #13916, #12771, #4569, #2288, #10174, #12692, #13680, #9117 ),
 .UNSPECIFIED., .F., .F.,
 ( 4, 2, 2, 2, 2, 2, 2, 2, 2, 4 ),
 ( 3.469446951953614189E-18, 0.0009765910691878101728, 0.001464886603781713308, 0.001953182138375616442, 0.002929773207563419243, 0.003906364276751221609, 0.004882955345939024409, 0.005859546415126826342, 0.006836137484314628275, 0.007812728553502431075 ),
 .UNSPECIFIED. ) ;
#2281=DIRECTION ( 'NONE',  ( 0.000000000000000000, 0.000000000000000000, -1.000000000000000000 ) ) ;
#2282=ORIENTED_EDGE ( 'NONE', *, *, #6282, .F. ) ;
#2286=ORIENTED_EDGE ( 'NONE', *, *, #3854, .F. ) ;
#2288=CARTESIAN_POINT ( 'NONE',  ( 32.92366211674485754, 95.48362627681292736, 15.74283067514923395 ) ) ;
#2291=DIRECTION ( 'NONE',  ( 1.000000000000000000, 0.000000000000000000, 0.000000000000000000 ) ) ;
#2305=CIRCLE ( 'NONE', #9079, 22.00000000000001421 ) ;
#2320=CARTESIAN_POINT ( 'NONE',  ( -8.076072847916480058, 62.48290708766281654, -19.99999999999999289 ) ) ;
#2323=ORIENTED_EDGE ( 'NONE', *, *, #2869, .T. ) ;
#2359=EDGE_CURVE ( 'NONE', #10315, #4701, #10405, .T. ) ;
#2362=CARTESIAN_POINT ( 'NONE',  ( -11.83526203526748333, 106.3435961965382290, 17.51264358390113784 ) ) ;
#2367=ORIENTED_EDGE ( 'NONE', *, *, #6018, .F. ) ;
#2375=VERTEX_POINT ( 'NONE', #9731 ) ;
#2380=DIRECTION ( 'NONE',  ( 0.000000000000000000, 0.000000000000000000, -1.000000000000000000 ) ) ;
#2385=CARTESIAN_POINT ( 'NONE',  ( -31.47058823529412663, 102.2673069760056563, -10.99999999999999645 ) ) ;
#2387=ORIENTED_EDGE ( 'NONE', *, *, #4129, .T. ) ;
#2414=CARTESIAN_POINT ( 'NONE',  ( -8.072319373765147077, 74.56485781596312279, -19.97535925451852989 ) ) ;
#2417=DIRECTION ( 'NONE',  ( 1.000000000000000000, 0.000000000000000000, 0.000000000000000000 ) ) ;
#2422=CIRCLE ( 'NONE', #11159, 5.000000000000000888 ) ;
#2436=CARTESIAN_POINT ( 'NONE',  ( 22.05882352941176094, 71.68269180561141241, 16.00000000000000000 ) ) ;
#2440=CARTESIAN_POINT ( 'NONE',  ( -12.23689275498546714, 106.2979809871390131, -16.60898801976832573 ) ) ;
#2447=VERTEX_POINT ( 'NONE', #14617 ) ;
#2452=LINE ( 'NONE', #4524, #8241 ) ;
#2457=ADVANCED_FACE ( 'NONE', ( #12403 ), #7457, .T. ) ;
#2461=CARTESIAN_POINT ( 'NONE',  ( 12.39897948556635754, 61.76783392443436327, 16.00000000000000000 ) ) ;
#2464=CIRCLE ( 'NONE', #12900, 7.500000000000001776 ) ;
#2468=CARTESIAN_POINT ( 'NONE',  ( 12.49999999999999645, 106.2673515243510991, 15.33083626825422741 ) ) ;
#2481=EDGE_CURVE ( 'NONE', #10943, #12827, #1856, .T. ) ;
#2493=DIRECTION ( 'NONE',  ( -1.000000000000000000, 0.000000000000000000, 0.000000000000000000 ) ) ;
#2494=ORIENTED_EDGE ( 'NONE', *, *, #4469, .F. ) ;
#2497=CARTESIAN_POINT ( 'NONE',  ( 5.204748896376250896E-15, 85.00000000000000000, 31.00000000000000000 ) ) ;
#2498=ORIENTED_EDGE ( 'NONE', *, *, #3771, .F. ) ;
#2500=AXIS2_PLACEMENT_3D ( 'NONE', #11397, #14104, #13674 ) ;
#2502=EDGE_LOOP ( 'NONE', ( #6535, #8024, #3119, #8972, #6519 ) ) ;
#2514=ORIENTED_EDGE ( 'NONE', *, *, #14240, .F. ) ;
#2517=AXIS2_PLACEMENT_3D ( 'NONE', #8968, #11342, #11700 ) ;
#2520=CARTESIAN_POINT ( 'NONE',  ( 8.915162460657667154, 94.58113943660329426, -19.80393736615727462 ) ) ;
#2521=DIRECTION ( 'NONE',  ( -0.000000000000000000, 0.000000000000000000, 1.000000000000000000 ) ) ;
#2524=AXIS2_PLACEMENT_3D ( 'NONE', #11645, #3668, #12703 ) ;
#2528=DIRECTION ( 'NONE',  ( -0.000000000000000000, -0.000000000000000000, 1.000000000000000000 ) ) ;
#2539=VECTOR ( 'NONE', #1334, 1000.000000000000000 ) ;
#2540=LINE ( 'NONE', #1553, #8387 ) ;
#2544=ORIENTED_EDGE ( 'NONE', *, *, #14530, .F. ) ;
#2551=AXIS2_PLACEMENT_3D ( 'NONE', #6927, #8075, #1176 ) ;
#2552=CARTESIAN_POINT ( 'NONE',  ( 10.00610186947451830, 106.5314655734665052, 19.33904518629107017 ) ) ;
#2562=DIRECTION ( 'NONE',  ( -1.000000000000000000, 0.000000000000000000, 0.000000000000000000 ) ) ;
#2564=CARTESIAN_POINT ( 'NONE',  ( 25.00000000000000000, 81.24038404635960831, -23.50000000000000000 ) ) ;
#2573=CARTESIAN_POINT ( 'NONE',  ( -25.00000000000000000, 81.24038404635962252, 23.50000000000000355 ) ) ;
#2574=DIRECTION ( 'NONE',  ( 0.9557692240748189016, 0.2941176470588237613, 0.000000000000000000 ) ) ;
#2585=CARTESIAN_POINT ( 'NONE',  ( 33.82975856321728969, 101.3925934381291256, -15.34957766734057927 ) ) ;
#2587=EDGE_CURVE ( 'NONE', #6805, #10315, #7981, .T. ) ;
#2592=B_SPLINE_CURVE_WITH_KNOTS ( 'NONE', 3,
 ( #5977, #14390, #5128, #2923, #1430, #10541, #3997, #9825, #12192, #10609 ),
 .UNSPECIFIED., .F., .F.,
 ( 4, 2, 2, 2, 4 ),
 ( 0.000000000000000000, 0.001711864931188370777, 0.003423729862376741553, 0.005135594793565112330, 0.006847459724753483107 ),
 .UNSPECIFIED. ) ;
#2600=CARTESIAN_POINT ( 'NONE',  ( -27.94117647058823550, 90.79807628710781842, -23.50000000000000000 ) ) ;
#2607=DIRECTION ( 'NONE',  ( 0.2941176470588234837, 0.9557692240748187906, 0.000000000000000000 ) ) ;
#2609=CARTESIAN_POINT ( 'NONE',  ( -31.95875033779847030, 102.1112180006092842, -13.22918226575833955 ) ) ;
#2618=VERTEX_POINT ( 'NONE', #12484 ) ;
#2619=AXIS2_PLACEMENT_3D ( 'NONE', #4922, #4696, #9383 ) ;
#2627=EDGE_LOOP ( 'NONE', ( #6115, #8990, #2494, #3096 ) ) ;
#2637=CARTESIAN_POINT ( 'NONE',  ( 0.000000000000000000, 0.000000000000000000, 16.00000000000000000 ) ) ;
#2657=CARTESIAN_POINT ( 'NONE',  ( 34.64620656398769682, 101.0151817716822933, -15.74933755401541902 ) ) ;
#2665=VECTOR ( 'NONE', #12343, 1000.000000000000000 ) ;
#2677=EDGE_CURVE ( 'NONE', #5269, #10950, #13666, .T. ) ;
#2680=CARTESIAN_POINT ( 'NONE',  ( -7.500000000000000888, 106.2673515243510991, 20.00000000000000000 ) ) ;
#2681=AXIS2_PLACEMENT_3D ( 'NONE', #1527, #6141, #11790 ) ;
#2687=CARTESIAN_POINT ( 'NONE',  ( -25.00000000000000000, 81.24038404635962252, 31.00000000000000000 ) ) ;
#2698=CARTESIAN_POINT ( 'NONE',  ( 22.05882352941176094, 71.68269180561141241, -16.00000000000000000 ) ) ;
#2707=DIRECTION ( 'NONE',  ( -1.000000000000000000, 0.000000000000000000, -0.000000000000000000 ) ) ;
#2720=CARTESIAN_POINT ( 'NONE',  ( -12.39897948556635754, 73.96800191783272282, 16.00000000000000000 ) ) ;
#2728=ORIENTED_EDGE ( 'NONE', *, *, #8981, .T. ) ;
#2731=VECTOR ( 'NONE', #13721, 1000.000000000000114 ) ;
#2736=EDGE_CURVE ( 'NONE', #11234, #6805, #4051, .T. ) ;
#2751=AXIS2_PLACEMENT_3D ( 'NONE', #13758, #2129, #14743 ) ;
#2756=CARTESIAN_POINT ( 'NONE',  ( 30.00000000000001066, 97.48846085563154418, -26.00000000000000000 ) ) ;
#2757=DIRECTION ( 'NONE',  ( 1.000000000000000000, 0.000000000000000000, 0.000000000000000000 ) ) ;
#2759=CARTESIAN_POINT ( 'NONE',  ( -31.47058823529412663, 102.2673069760056563, -10.99999999999999645 ) ) ;
#2767=AXIS2_PLACEMENT_3D ( 'NONE', #13469, #7613, #12556 ) ;
#2769=VECTOR ( 'NONE', #778, 1000.000000000000000 ) ;
#2772=VERTEX_POINT ( 'NONE', #5252 ) ;
#2792=ORIENTED_EDGE ( 'NONE', *, *, #5931, .T. ) ;
#2799=AXIS2_PLACEMENT_3D ( 'NONE', #4648, #11576, #2291 ) ;
#2810=CARTESIAN_POINT ( 'NONE',  ( -31.32379180359345838, 96.02017129613334134, 14.76790389961145600 ) ) ;
#2817=LINE ( 'NONE', #4875, #6994 ) ;
#2829=CARTESIAN_POINT ( 'NONE',  ( 29.70588235294119173, 96.53269163155674448, -10.99999999999999645 ) ) ;
#2843=DIRECTION ( 'NONE',  ( 1.000000000000000000, 0.000000000000000000, 0.000000000000000000 ) ) ;
#2854=CARTESIAN_POINT ( 'NONE',  ( -29.73684566822694464, 96.52317875358642141, -11.65491793965443001 ) ) ;
#2859=DIRECTION ( 'NONE',  ( 0.000000000000000000, 0.000000000000000000, -1.000000000000000000 ) ) ;
#2869=EDGE_CURVE ( 'NONE', #14637, #14691, #8945, .T. ) ;
#2871=DIRECTION ( 'NONE',  ( 0.000000000000000000, -0.000000000000000000, -1.000000000000000000 ) ) ;
#2875=ADVANCED_FACE ( 'NONE', ( #4422 ), #7346, .T. ) ;
#2882=CARTESIAN_POINT ( 'NONE',  ( 35.00000000000000000, 81.24038404635960831, -16.00000000000000000 ) ) ;
#2891=CARTESIAN_POINT ( 'NONE',  ( 30.19044911324211711, 96.38232397946876517, -13.21859331841448792 ) ) ;
#2894=CARTESIAN_POINT ( 'NONE',  ( -12.50000000000000000, 40.62019202317981126, -23.50000000000000000 ) ) ;
#2898=DIRECTION ( 'NONE',  ( -0.000000000000000000, -0.000000000000000000, 1.000000000000000000 ) ) ;
#2903=EDGE_CURVE ( 'NONE', #14727, #2447, #12694, .T. ) ;
#2916=AXIS2_PLACEMENT_3D ( 'NONE', #2573, #373, #14262 ) ;
#2918=EDGE_CURVE ( 'NONE', #14637, #7984, #82, .T. ) ;
#2922=EDGE_CURVE ( 'NONE', #5730, #14727, #7736, .T. ) ;
#2923=CARTESIAN_POINT ( 'NONE',  ( -9.718176292668218252, 74.36971601906103047, 19.51774219187060311 ) ) ;
#2929=CIRCLE ( 'NONE', #2681, 68.00000000000000000 ) ;
#2938=ADVANCED_BREP_SHAPE_REPRESENTATION ( '', ( #8964, #5108 ), #14072 ) ;
#2946=DIRECTION ( 'NONE',  ( -0.000000000000000000, -0.000000000000000000, -1.000000000000000000 ) ) ;
#2948=CARTESIAN_POINT ( 'NONE',  ( -33.08545438203827871, 101.7020459634811118, 14.77901645503695427 ) ) ;
#2978=ORIENTED_EDGE ( 'NONE', *, *, #506, .F. ) ;
#2981=CARTESIAN_POINT ( 'NONE',  ( 9.716053034936797062, 106.5583837859906566, 19.49385781195229583 ) ) ;
#2986=CARTESIAN_POINT ( 'NONE',  ( -11.08614924580848360, 94.35111528408442894, 18.49588680517285155 ) ) ;
#2991=CIRCLE ( 'NONE', #1782, 10.00000000000000355 ) ;
#3001=CARTESIAN_POINT ( 'NONE',  ( 31.47058823529413374, 102.2673069760056563, -26.00000000000000000 ) ) ;
#3002=FACE_OUTER_BOUND ( 'NONE', #10381, .T. ) ;
#3005=ORIENTED_EDGE ( 'NONE', *, *, #8971, .F. ) ;
#3017=EDGE_CURVE ( 'NONE', #3168, #5730, #2991, .T. ) ;
#3018=ORIENTED_EDGE ( 'NONE', *, *, #7238, .F. ) ;
#3021=EDGE_CURVE ( 'NONE', #2375, #14939, #11990, .T. ) ;
#3026=( NAMED_UNIT ( * ) PLANE_ANGLE_UNIT ( ) SI_UNIT ( $, .RADIAN. ) );
#3031=CARTESIAN_POINT ( 'NONE',  ( -32.45028783375101256, 101.9412720646926260, 14.06019896931749358 ) ) ;
#3038=B_SPLINE_CURVE_WITH_KNOTS ( 'NONE', 3,
 ( #5522, #13560, #10142, #10077 ),
 .UNSPECIFIED., .F., .F.,
 ( 4, 4 ),
 ( 0.000000000000000000, 0.001005167940839973807 ),
 .UNSPECIFIED. ) ;
#3040=CARTESIAN_POINT ( 'NONE',  ( -29.95202887341199371, 96.45668229681565720, 12.61733007774791915 ) ) ;
#3045=UNCERTAINTY_MEASURE_WITH_UNIT (LENGTH_MEASURE( 1.000000000000000082E-05 ), #9128, 'distance_accuracy_value', 'NONE');
#3057=ORIENTED_EDGE ( 'NONE', *, *, #13026, .F. ) ;
#3060=DIRECTION ( 'NONE',  ( -0.000000000000000000, -0.000000000000000000, 1.000000000000000000 ) ) ;
#3066=CARTESIAN_POINT ( 'NONE',  ( -12.50000000000000000, 100.2235002382176248, -15.00000000000000000 ) ) ;
#3070=DIRECTION ( 'NONE',  ( -0.000000000000000000, 1.000000000000000000, -0.000000000000000000 ) ) ;
#3077=VECTOR ( 'NONE', #8143, 1000.000000000000000 ) ;
#3078=EDGE_CURVE ( 'NONE', #14649, #944, #9515, .T. ) ;
#3080=CARTESIAN_POINT ( 'NONE',  ( -12.39897948556635754, 94.18739463280904545, 16.00000000000000000 ) ) ;
#3091=CARTESIAN_POINT ( 'NONE',  ( 33.32958405265417667, 101.6044047647129958, 14.99207720203049199 ) ) ;
#3096=ORIENTED_EDGE ( 'NONE', *, *, #14155, .F. ) ;
#3101=LINE ( 'NONE', #13733, #7179 ) ;
#3104=CARTESIAN_POINT ( 'NONE',  ( -31.77701906416544730, 102.1706497334997863, 12.77113345645743969 ) ) ;
#3107=ORIENTED_EDGE ( 'NONE', *, *, #4805, .F. ) ;
#3111=FACE_OUTER_BOUND ( 'NONE', #643, .T. ) ;
#3119=ORIENTED_EDGE ( 'NONE', *, *, #5188, .T. ) ;
#3126=CARTESIAN_POINT ( 'NONE',  ( -12.50000000000000000, 106.2673515243510991, -15.00000000000000000 ) ) ;
#3127=VERTEX_POINT ( 'NONE', #10677 ) ;
#3139=EDGE_CURVE ( 'NONE', #4446, #259, #1543, .T. ) ;
#3143=CARTESIAN_POINT ( 'NONE',  ( 12.05137958362237960, 94.23255994477487718, -17.08976535968791310 ) ) ;
#3145=DIRECTION ( 'NONE',  ( -1.000000000000000000, 0.000000000000000000, 0.000000000000000000 ) ) ;
#3150=CIRCLE ( 'NONE', #11640, 22.00000000000000000 ) ;
#3152=DIRECTION ( 'NONE',  ( 0.000000000000000000, 0.000000000000000000, -1.000000000000000000 ) ) ;
#3155=CARTESIAN_POINT ( 'NONE',  ( 11.46932393819253804, 106.3836852522821488, -18.05815993169796130 ) ) ;
#3160=ORIENTED_EDGE ( 'NONE', *, *, #1928, .T. ) ;
#3164=CARTESIAN_POINT ( 'NONE',  ( 34.09969740539978744, 101.2725728942521073, 15.50446122302712304 ) ) ;
#3167=EDGE_LOOP ( 'NONE', ( #7347, #9473 ) ) ;
#3168=VERTEX_POINT ( 'NONE', #4158 ) ;
#3173=PLANE ( 'NONE',  #7579 ) ;
#3174=FILL_AREA_STYLE ('',( #12438 ) ) ;
#3182=AXIS2_PLACEMENT_3D ( 'NONE', #10973, #8683, #575 ) ;
#3193=VECTOR ( 'NONE', #14768, 1000.000000000000000 ) ;
#3196=CARTESIAN_POINT ( 'NONE',  ( 12.28299983316190946, 61.79111512501306436, 16.56818193787249527 ) ) ;
#3212=VECTOR ( 'NONE', #13025, 1000.000000000000000 ) ;
#3213=FACE_BOUND ( 'NONE', #4830, .T. ) ;
#3221=AXIS2_PLACEMENT_3D ( 'NONE', #4064, #12335, #3145 ) ;
#3226=PLANE ( 'NONE',  #3270 ) ;
#3234=ORIENTED_EDGE ( 'NONE', *, *, #979, .F. ) ;
#3242=EDGE_CURVE ( 'NONE', #13289, #337, #11214, .T. ) ;
#3258=ORIENTED_EDGE ( 'NONE', *, *, #73, .F. ) ;
#3270=AXIS2_PLACEMENT_3D ( 'NONE', #7844, #10125, #806 ) ;
#3275=CARTESIAN_POINT ( 'NONE',  ( 12.39897948556635754, 61.76783392443436327, 16.00000000000000000 ) ) ;
#3276=CARTESIAN_POINT ( 'NONE',  ( 18.52941176470587692, 60.21346111671358159, 31.00000000000000000 ) ) ;
#3280=CARTESIAN_POINT ( 'NONE',  ( 29.73684566822694464, 96.52317875358639299, 11.65491793965443357 ) ) ;
#3285=CARTESIAN_POINT ( 'NONE',  ( -11.26223186129995391, 106.4059016791561447, 18.30934846123060922 ) ) ;
#3287=EDGE_CURVE ( 'NONE', #5421, #7249, #4918, .T. ) ;
#3295=ORIENTED_EDGE ( 'NONE', *, *, #11069, .F. ) ;
#3316=CARTESIAN_POINT ( 'NONE',  ( 35.79345569434273244, 100.4135791079097544, 15.99999999999999645 ) ) ;
#3318=ORIENTED_EDGE ( 'NONE', *, *, #9787, .F. ) ;
#3319=ORIENTED_EDGE ( 'NONE', *, *, #4805, .T. ) ;
#3323=DIRECTION ( 'NONE',  ( 1.000000000000000000, 0.000000000000000000, 0.000000000000000000 ) ) ;
#3325=DIRECTION ( 'NONE',  ( -0.000000000000000000, -0.000000000000000000, 1.000000000000000000 ) ) ;
#3327=CARTESIAN_POINT ( 'NONE',  ( -12.39897948556635754, 61.76783392443436327, -16.00000000000000000 ) ) ;
#3331=EDGE_CURVE ( 'NONE', #5203, #337, #8083, .T. ) ;
#3334=ORIENTED_EDGE ( 'NONE', *, *, #4129, .F. ) ;
#3336=CYLINDRICAL_SURFACE ( 'NONE', #3909, 7.500000000000001776 ) ;
#3338=CARTESIAN_POINT ( 'NONE',  ( -25.00000000000000000, 81.24038404635962252, -23.50000000000000000 ) ) ;
#3342=EDGE_LOOP ( 'NONE', ( #8519, #2544, #13031, #3005, #11209, #8955 ) ) ;
#3351=CARTESIAN_POINT ( 'NONE',  ( 29.70588235294119528, 96.53269163155674448, 11.33021710499463985 ) ) ;
#3352=AXIS2_PLACEMENT_3D ( 'NONE', #7097, #13891, #2562 ) ;
#3355=CARTESIAN_POINT ( 'NONE',  ( -9.260566377415146988, 106.5986160369160416, 19.68264575353695989 ) ) ;
#3356=CYLINDRICAL_SURFACE ( 'NONE', #6593, 75.00000000000001421 ) ;
#3366=DIRECTION ( 'NONE',  ( -0.2941176470588243164, -0.9557692240748185686, -0.000000000000000000 ) ) ;
#3368=ORIENTED_EDGE ( 'NONE', *, *, #7369, .F. ) ;
#3375=ORIENTED_EDGE ( 'NONE', *, *, #14454, .F. ) ;
#3378=CARTESIAN_POINT ( 'NONE',  ( -15.11621636258860946, 32.12188890498260463, -16.00000000000000000 ) ) ;
#3382=ORIENTED_EDGE ( 'NONE', *, *, #1535, .F. ) ;
#3383=AXIS2_PLACEMENT_3D ( 'NONE', #14740, #6358, #14590 ) ;
#3388=CARTESIAN_POINT ( 'NONE',  ( 9.448652591187071792, 74.40292581525912397, 19.61336856585178623 ) ) ;
#3390=CIRCLE ( 'NONE', #13096, 4.999999999999995559 ) ;
#3392=CARTESIAN_POINT ( 'NONE',  ( 0.000000000000000000, 0.000000000000000000, -23.50000000000000000 ) ) ;
#3395=LINE ( 'NONE', #3700, #14697 ) ;
#3396=AXIS2_PLACEMENT_3D ( 'NONE', #8894, #1843, #13461 ) ;
#3401=DIRECTION ( 'NONE',  ( -0.000000000000000000, -0.000000000000000000, -1.000000000000000000 ) ) ;
#3420=CARTESIAN_POINT ( 'NONE',  ( 27.94117647058824616, 90.79807628710781842, 16.00000000000000000 ) ) ;
#3427=CARTESIAN_POINT ( 'NONE',  ( 25.00000000000000000, 81.24038404635960831, 16.00000000000000000 ) ) ;
#3436=CIRCLE ( 'NONE', #13612, 68.00000000000000000 ) ;
#3459=ORIENTED_EDGE ( 'NONE', *, *, #15021, .T. ) ;
#3468=CARTESIAN_POINT ( 'NONE',  ( 10.44112439181167495, 74.26999561062542909, 19.05342973219118363 ) ) ;
#3469=AXIS2_PLACEMENT_3D ( 'NONE', #7915, #5716, #11646 ) ;
#3472=SURFACE_STYLE_FILL_AREA ( #3174 ) ;
#3477=EDGE_CURVE ( 'NONE', #14956, #14203, #10293, .T. ) ;
#3483=AXIS2_PLACEMENT_3D ( 'NONE', #5804, #3325, #4686 ) ;
#3508=CARTESIAN_POINT ( 'NONE',  ( 30.18932686484986760, 96.38267619380722806, 13.21651853314491198 ) ) ;
#3509=ORIENTED_EDGE ( 'NONE', *, *, #8652, .T. ) ;
#3516=CIRCLE ( 'NONE', #9320, 7.500000000000001776 ) ;
#3519=PLANE ( 'NONE',  #6327 ) ;
#3525=EDGE_CURVE ( 'NONE', #10333, #13430, #3989, .T. ) ;
#3532=VERTEX_POINT ( 'NONE', #1482 ) ;
#3535=ADVANCED_FACE ( 'NONE', ( #14237 ), #14083, .T. ) ;
#3537=CARTESIAN_POINT ( 'NONE',  ( 30.00000000000001066, 97.48846085563154418, -31.00000000000000000 ) ) ;
#3540=VERTEX_POINT ( 'NONE', #4902 ) ;
#3543=EDGE_CURVE ( 'NONE', #4701, #4832, #6019, .T. ) ;
#3572=CARTESIAN_POINT ( 'NONE',  ( -10.44112439181167495, 74.26999561062542909, -19.05342973219118008 ) ) ;
#3582=CARTESIAN_POINT ( 'NONE',  ( 30.00974697327758989, 96.43868009418279996, 12.76250177908514516 ) ) ;
#3589=CYLINDRICAL_SURFACE ( 'NONE', #14781, 10.00000000000000178 ) ;
#3590=DIRECTION ( 'NONE',  ( 1.000000000000000000, 0.000000000000000000, 0.000000000000000000 ) ) ;
#3596=B_SPLINE_CURVE_WITH_KNOTS ( 'NONE', 3,
 ( #12176, #11878, #5264, #12101, #6382, #9646, #1693, #6300, #7380, #13164, #335, #3760, #6233, #8381, #2609, #411, #4972, #9584, #5111, #2759 ),
 .UNSPECIFIED., .F., .F.,
 ( 4, 2, 2, 2, 2, 2, 2, 2, 2, 4 ),
 ( 1.430489624538199204E-17, 0.0009816351435713611961, 0.001472452715357042662, 0.001963270287142724127, 0.002944905430714070578, 0.003926540574285417029, 0.004908175717856764347, 0.005889810861428110798, 0.006871446004999457249, 0.007853081148570804568 ),
 .UNSPECIFIED. ) ;
#3605=EDGE_CURVE ( 'NONE', #8733, #4832, #2003, .T. ) ;
#3616=ORIENTED_EDGE ( 'NONE', *, *, #979, .T. ) ;
#3618=CARTESIAN_POINT ( 'NONE',  ( 11.83867104060235853, 106.3432143034624033, 17.50653253748099303 ) ) ;
#3624=EDGE_LOOP ( 'NONE', ( #1137, #10558, #14843, #4037 ) ) ;
#3628=CARTESIAN_POINT ( 'NONE',  ( 7.500000000000000000, 62.55197838597913318, 20.00000000000000000 ) ) ;
#3630=VERTEX_POINT ( 'NONE', #6240 ) ;
#3638=EDGE_LOOP ( 'NONE', ( #7398, #14292 ) ) ;
#3639=CARTESIAN_POINT ( 'NONE',  ( -30.00000000000000711, 97.48846085563154418, 26.00000000000000000 ) ) ;
#3645=CIRCLE ( 'NONE', #1937, 10.00000000000000178 ) ;
#3647=CIRCLE ( 'NONE', #12135, 4.999999999999994671 ) ;
#3656=DIRECTION ( 'NONE',  ( -1.000000000000000000, 0.000000000000000000, -0.000000000000000000 ) ) ;
#3667=CARTESIAN_POINT ( 'NONE',  ( -9.115592515563381681, 106.6114291000284027, -19.74294316973679742 ) ) ;
#3668=DIRECTION ( 'NONE',  ( -0.000000000000000000, -0.000000000000000000, -1.000000000000000000 ) ) ;
#3678=LINE ( 'NONE', #4588, #7751 ) ;
#3680=AXIS2_PLACEMENT_3D ( 'NONE', #9648, #478, #7524 ) ;
#3691=EDGE_CURVE ( 'NONE', #5730, #4479, #10252, .T. ) ;
#3696=CARTESIAN_POINT ( 'NONE',  ( 10.80358476664835266, 106.4534462909512769, 18.76728514983858531 ) ) ;
#3697=CARTESIAN_POINT ( 'NONE',  ( 5.204748896376250896E-15, 85.00000000000000000, 31.00000000000000000 ) ) ;
#3700=CARTESIAN_POINT ( 'NONE',  ( 12.50000000000000000, 61.74746958378133144, -15.00000000000000355 ) ) ;
#3701=ORIENTED_EDGE ( 'NONE', *, *, #14984, .F. ) ;
#3714=ORIENTED_EDGE ( 'NONE', *, *, #5374, .F. ) ;
#3723=CARTESIAN_POINT ( 'NONE',  ( -7.787661217455939422, 74.59514674284385194, -20.00000000000000000 ) ) ;
#3727=FACE_OUTER_BOUND ( 'NONE', #11669, .T. ) ;
#3731=ORIENTED_EDGE ( 'NONE', *, *, #14454, .T. ) ;
#3733=CARTESIAN_POINT ( 'NONE',  ( 12.39897948556635576, 94.18739463280904545, 16.00000000000000000 ) ) ;
#3734=ORIENTED_EDGE ( 'NONE', *, *, #10885, .T. ) ;
#3760=CARTESIAN_POINT ( 'NONE',  ( -32.65306121041741250, 101.8676703390407141, -14.32076206672372543 ) ) ;
#3771=EDGE_CURVE ( 'NONE', #14203, #12897, #10964, .T. ) ;
#3772=AXIS2_PLACEMENT_3D ( 'NONE', #12929, #5935, #6003 ) ;
#3776=CARTESIAN_POINT ( 'NONE',  ( 7.829984960685308693, 106.7136390683880336, 20.00000000000000355 ) ) ;
#3781=DIRECTION ( 'NONE',  ( -0.000000000000000000, -0.000000000000000000, 1.000000000000000000 ) ) ;
#3785=ORIENTED_EDGE ( 'NONE', *, *, #2124, .F. ) ;
#3794=ORIENTED_EDGE ( 'NONE', *, *, #3605, .T. ) ;
#3796=DIRECTION ( 'NONE',  ( -0.2941176470588241498, 0.9557692240748186796, 0.000000000000000000 ) ) ;
#3807=EDGE_LOOP ( 'NONE', ( #4917, #12571, #7703, #10159 ) ) ;
#3813=CARTESIAN_POINT ( 'NONE',  ( -7.500000000000000888, 62.55197838597913318, -20.00000000000000000 ) ) ;
#3817=DIRECTION ( 'NONE',  ( 0.000000000000000000, -1.000000000000000000, -0.000000000000000000 ) ) ;
#3834=ORIENTED_EDGE ( 'NONE', *, *, #8234, .F. ) ;
#3839=EDGE_CURVE ( 'NONE', #4879, #3532, #10980, .T. ) ;
#3846=DIRECTION ( 'NONE',  ( -0.000000000000000000, -0.000000000000000000, 1.000000000000000000 ) ) ;
#3848=PLANE ( 'NONE',  #13722 ) ;
#3849=ORIENTED_EDGE ( 'NONE', *, *, #10637, .F. ) ;
#3854=EDGE_CURVE ( 'NONE', #12353, #6653, #6601, .T. ) ;
#3892=CARTESIAN_POINT ( 'NONE',  ( -12.37198577373457553, 106.2823362334109447, -16.13593661559556836 ) ) ;
#3893=CYLINDRICAL_SURFACE ( 'NONE', #2018, 5.000000000000001776 ) ;
#3901=AXIS2_PLACEMENT_3D ( 'NONE', #13800, #12513, #11374 ) ;
#3908=CARTESIAN_POINT ( 'NONE',  ( -7.500000000000000888, 94.70348462437907244, 20.00000000000000000 ) ) ;
#3909=AXIS2_PLACEMENT_3D ( 'NONE', #5757, #8258, #5826 ) ;
#3919=AXIS2_PLACEMENT_3D ( 'NONE', #7800, #2871, #1811 ) ;
#3921=ORIENTED_EDGE ( 'NONE', *, *, #532, .T. ) ;
#3923=CARTESIAN_POINT ( 'NONE',  ( 10.19763225997207634, 62.16969414240131897, -19.21937000502254023 ) ) ;
#3924=CIRCLE ( 'NONE', #12894, 10.00000000000000355 ) ;
#3948=ORIENTED_EDGE ( 'NONE', *, *, #2165, .F. ) ;
#3954=CARTESIAN_POINT ( 'NONE',  ( 31.50188001269984994, 102.2577498558884486, -11.65822132526735899 ) ) ;
#3956=CARTESIAN_POINT ( 'NONE',  ( 5.204748896376250896E-15, 85.00000000000000000, 46.00000000000000000 ) ) ;
#3964=ORIENTED_EDGE ( 'NONE', *, *, #13412, .T. ) ;
#3969=ORIENTED_EDGE ( 'NONE', *, *, #10762, .T. ) ;
#3970=CARTESIAN_POINT ( 'NONE',  ( 30.88479107129467849, 96.16227383530471684, -14.30703002621669562 ) ) ;
#3973=ORIENTED_EDGE ( 'NONE', *, *, #8971, .T. ) ;
#3986=CARTESIAN_POINT ( 'NONE',  ( 25.00000000000000000, 81.24038404635960831, -31.00000000000000000 ) ) ;
#3987=UNCERTAINTY_MEASURE_WITH_UNIT (LENGTH_MEASURE( 1.000000000000000082E-05 ), #13732, 'distance_accuracy_value', 'NONE');
#3989=LINE ( 'NONE', #13097, #3212 ) ;
#3997=CARTESIAN_POINT ( 'NONE',  ( -11.47770164139309301, 74.11716252799973859, 18.08381726540838486 ) ) ;
#4003=AXIS2_PLACEMENT_3D ( 'NONE', #223, #9555, #308 ) ;
#4005=ORIENTED_EDGE ( 'NONE', *, *, #5698, .T. ) ;
#4006=ADVANCED_FACE ( 'NONE', ( #7063 ), #1617, .T. ) ;
#4010=VERTEX_POINT ( 'NONE', #2600 ) ;
#4012=CYLINDRICAL_SURFACE ( 'NONE', #8584, 63.00000000000000000 ) ;
#4014=ORIENTED_EDGE ( 'NONE', *, *, #4030, .T. ) ;
#4025=B_SPLINE_CURVE_WITH_KNOTS ( 'NONE', 3,
 ( #5486, #5408, #14680, #10109, #11406, #9265, #6910, #10626, #9187, #8131, #4506, #13836, #4647, #6833 ),
 .UNSPECIFIED., .F., .F.,
 ( 4, 2, 2, 2, 2, 2, 4 ),
 ( 0.000000000000000000, 0.001716022237784528602, 0.002574033356676790844, 0.003432044475569052868, 0.004290055594461314459, 0.005148066713353576483, 0.006864088951138102267 ),
 .UNSPECIFIED. ) ;
#4027=DIRECTION ( 'NONE',  ( 0.000000000000000000, 0.000000000000000000, 1.000000000000000000 ) ) ;
#4030=EDGE_CURVE ( 'NONE', #1777, #14691, #14194, .T. ) ;
#4032=CARTESIAN_POINT ( 'NONE',  ( 34.09759333678488247, 101.2734996710205593, -15.50321023462187853 ) ) ;
#4035=DIRECTION ( 'NONE',  ( -0.000000000000000000, -0.000000000000000000, 1.000000000000000000 ) ) ;
#4037=ORIENTED_EDGE ( 'NONE', *, *, #7238, .T. ) ;
#4047=EDGE_CURVE ( 'NONE', #5260, #13905, #7142, .T. ) ;
#4048=ORIENTED_EDGE ( 'NONE', *, *, #7590, .T. ) ;
#4051=CIRCLE ( 'NONE', #14958, 63.00000000000000000 ) ;
#4055=CARTESIAN_POINT ( 'NONE',  ( 27.94117647058824616, 90.79807628710781842, -23.50000000000000000 ) ) ;
#4059=CARTESIAN_POINT ( 'NONE',  ( 47.00000000000001421, 81.24038404635960831, -26.00000000000000000 ) ) ;
#4061=ORIENTED_EDGE ( 'NONE', *, *, #5695, .F. ) ;
#4062=CARTESIAN_POINT ( 'NONE',  ( 8.635299310232698033, 74.50321615228340022, -19.90320263233617482 ) ) ;
#4064=CARTESIAN_POINT ( 'NONE',  ( 25.00000000000000000, 81.24038404635960831, -23.50000000000000000 ) ) ;
#4072=DIRECTION ( 'NONE',  ( -1.000000000000000000, 0.000000000000000000, 0.000000000000000000 ) ) ;
#4074=CLOSED_SHELL ( 'NONE', ( #8336, #14138, #10257, #10372, #4553, #7136, #597, #835, #8465, #320, #13179, #7400, #960, #11848, #6091, #6800, #220, #2032, #12947, #1976, #9516, #12883, #5963, #10553, #4920, #12024, #9166, #69, #4126, #6176, #3535, #12244, #14526, #10367, #7087, #720, #12936, #4006, #10793, #11373, #12845, #12892, #155, #10610, #5326, #7834, #8116, #5518, #4497, #2875, #10848, #8994, #11217, #1203, #2457, #12532, #13724, #12022, #11169, #9696, #7817, #14483, #6854, #14432, #1800 ) ) ;
#4077=CARTESIAN_POINT ( 'NONE',  ( -34.13789039812932913, 95.05637002121839885, -16.00000000000000355 ) ) ;
#4084=B_SPLINE_CURVE_WITH_KNOTS ( 'NONE', 3,
 ( #865, #10111, #13601, #10178, #10264, #7826, #705, #14827, #4350, #12471 ),
 .UNSPECIFIED., .F., .F.,
 ( 4, 2, 2, 2, 4 ),
 ( 0.000000000000000000, 0.001708674401391109456, 0.003417348802782218913, 0.005126023204173327935, 0.006834697605564437825 ),
 .UNSPECIFIED. ) ;
#4092=ORIENTED_EDGE ( 'NONE', *, *, #15021, .F. ) ;
#4100=DIRECTION ( 'NONE',  ( 1.000000000000000000, -1.332267629550187849E-14, 0.000000000000000000 ) ) ;
#4102=DIRECTION ( 'NONE',  ( 0.000000000000000000, -1.000000000000000000, 0.000000000000000000 ) ) ;
#4105=ORIENTED_EDGE ( 'NONE', *, *, #14155, .T. ) ;
#4107=CARTESIAN_POINT ( 'NONE',  ( 0.000000000000000000, 0.000000000000000000, -79.80561291909842225 ) ) ;
#4110=TOROIDAL_SURFACE ( 'NONE', #8700, 68.00000000000000000, 5.000000000000000000 ) ;
#4113=FACE_OUTER_BOUND ( 'NONE', #9321, .T. ) ;
#4124=AXIS2_PLACEMENT_3D ( 'NONE', #11846, #12982, #13208 ) ;
#4126=ADVANCED_FACE ( 'NONE', ( #4113 ), #6367, .F. ) ;
#4129=EDGE_CURVE ( 'NONE', #1495, #13289, #11507, .T. ) ;
#4131=CARTESIAN_POINT ( 'NONE',  ( -11.92530613726453659, 94.24865542230074311, 17.34466199971670264 ) ) ;
#4133=CARTESIAN_POINT ( 'NONE',  ( 8.075966873893682063, 74.56617093413656505, -19.99999999999999645 ) ) ;
#4146=CARTESIAN_POINT ( 'NONE',  ( 5.000000000000007105, 85.00000000000000000, 46.00000000000000000 ) ) ;
#4148=CARTESIAN_POINT ( 'NONE',  ( 7.500000000000000888, 62.55197838597913318, -20.00000000000000000 ) ) ;
#4151=ORIENTED_EDGE ( 'NONE', *, *, #15022, .F. ) ;
#4157=EDGE_CURVE ( 'NONE', #8172, #14105, #1341, .T. ) ;
#4158=CARTESIAN_POINT ( 'NONE',  ( 27.94117647058824616, 90.79807628710781842, -23.50000000000000000 ) ) ;
#4165=TOROIDAL_SURFACE ( 'NONE', #13853, 17.00000000000000000, 5.000000000000000000 ) ;
#4166=ORIENTED_EDGE ( 'NONE', *, *, #10007, .F. ) ;
#4180=EDGE_CURVE ( 'NONE', #15011, #9955, #12980, .T. ) ;
#4184=CARTESIAN_POINT ( 'NONE',  ( -34.13789339514570287, 95.05636893381519315, 15.99999999999999645 ) ) ;
#4186=CYLINDRICAL_SURFACE ( 'NONE', #7774, 5.000000000000001776 ) ;
#4194=VECTOR ( 'NONE', #5045, 1000.000000000000000 ) ;
#4198=VERTEX_POINT ( 'NONE', #7819 ) ;
#4216=AXIS2_PLACEMENT_3D ( 'NONE', #7815, #6675, #14894 ) ;
#4235=DIRECTION ( 'NONE',  ( 0.000000000000000000, 0.000000000000000000, 1.000000000000000000 ) ) ;
#4236=CARTESIAN_POINT ( 'NONE',  ( 32.10716661655239790, 102.0615849490105376, 13.52016324361725275 ) ) ;
#4240=ORIENTED_EDGE ( 'NONE', *, *, #3017, .F. ) ;
#4249=ORIENTED_EDGE ( 'NONE', *, *, #902, .T. ) ;
#4251=CARTESIAN_POINT ( 'NONE',  ( -31.50188001269984284, 102.2577498558884628, 11.65822132526736432 ) ) ;
#4260=DIRECTION ( 'NONE',  ( -0.000000000000000000, 0.000000000000000000, 1.000000000000000000 ) ) ;
#4267=CIRCLE ( 'NONE', #1595, 10.00000000000000178 ) ;
#4268=FACE_OUTER_BOUND ( 'NONE', #6304, .T. ) ;
#4274=CARTESIAN_POINT ( 'NONE',  ( 0.000000000000000000, 0.000000000000000000, -20.00000000000000000 ) ) ;
#4279=CARTESIAN_POINT ( 'NONE',  ( 12.39897948556635576, 73.96800191783272282, 16.00000000000000000 ) ) ;
#4294=CARTESIAN_POINT ( 'NONE',  ( -12.50000000000000000, 59.24038404635959409, -20.00000000000000000 ) ) ;
#4304=CARTESIAN_POINT ( 'NONE',  ( 12.46747951117848707, 106.2711918341631900, -15.65812229356676077 ) ) ;
#4325=ORIENTED_EDGE ( 'NONE', *, *, #2272, .T. ) ;
#4334=CARTESIAN_POINT ( 'NONE',  ( 7.500000000000000888, 74.62405778299650194, -20.00000000000000000 ) ) ;
#4350=CARTESIAN_POINT ( 'NONE',  ( -12.28362713749409529, 94.20257980066446635, -16.56510878681792320 ) ) ;
#4359=CARTESIAN_POINT ( 'NONE',  ( 10.20439220990035878, 94.45068983291282905, -19.21516791372541988 ) ) ;
#4365=ORIENTED_EDGE ( 'NONE', *, *, #4416, .F. ) ;
#4372=ORIENTED_EDGE ( 'NONE', *, *, #2359, .F. ) ;
#4373=CARTESIAN_POINT ( 'NONE',  ( 11.26223186129995923, 106.4059016791561731, -18.30934846123061632 ) ) ;
#4387=ORIENTED_EDGE ( 'NONE', *, *, #2869, .F. ) ;
#4405=ORIENTED_EDGE ( 'NONE', *, *, #13785, .T. ) ;
#4407=EDGE_CURVE ( 'NONE', #8663, #4528, #8380, .T. ) ;
#4413=CIRCLE ( 'NONE', #3680, 75.00000000000001421 ) ;
#4414=DIRECTION ( 'NONE',  ( 0.2941176470588238723, -0.9557692240748189016, 0.000000000000000000 ) ) ;
#4416=EDGE_CURVE ( 'NONE', #1158, #11234, #6433, .T. ) ;
#4419=ORIENTED_EDGE ( 'NONE', *, *, #3477, .T. ) ;
#4422=FACE_OUTER_BOUND ( 'NONE', #2039, .T. ) ;
#4427=EDGE_CURVE ( 'NONE', #10315, #1158, #10322, .T. ) ;
#4434=DIRECTION ( 'NONE',  ( 0.000000000000000000, 0.000000000000000000, 1.000000000000000000 ) ) ;
#4440=CARTESIAN_POINT ( 'NONE',  ( 30.00000000000000355, 97.48846085563152997, 26.00000000000000000 ) ) ;
#4446=VERTEX_POINT ( 'NONE', #9854 ) ;
#4450=AXIS2_PLACEMENT_3D ( 'NONE', #14946, #4763, #14867 ) ;
#4464=ORIENTED_EDGE ( 'NONE', *, *, #2922, .F. ) ;
#4465=ORIENTED_EDGE ( 'NONE', *, *, #4030, .F. ) ;
#4469=EDGE_CURVE ( 'NONE', #14546, #12897, #11118, .T. ) ;
#4473=CIRCLE ( 'NONE', #6149, 17.00000000000000000 ) ;
#4479=VERTEX_POINT ( 'NONE', #14655 ) ;
#4483=TOROIDAL_SURFACE ( 'NONE', #14411, 17.00000000000000000, 5.000000000000000000 ) ;
#4492=EDGE_LOOP ( 'NONE', ( #3057, #12469, #5074, #3734 ) ) ;
#4496=AXIS2_PLACEMENT_3D ( 'NONE', #11855, #1448, #10783 ) ;
#4497=ADVANCED_FACE ( 'NONE', ( #3111 ), #13976, .T. ) ;
#4506=CARTESIAN_POINT ( 'NONE',  ( -9.442781676091987819, 62.28890912541181990, 19.61600713740890001 ) ) ;
#4510=CARTESIAN_POINT ( 'NONE',  ( 7.500000000000000000, 61.74746958378133144, 20.00000000000000000 ) ) ;
#4511=DIRECTION ( 'NONE',  ( 0.000000000000000000, 0.000000000000000000, -1.000000000000000000 ) ) ;
#4524=CARTESIAN_POINT ( 'NONE',  ( 35.00000000000000000, 81.24038404635960831, 13.50000000000000533 ) ) ;
#4528=VERTEX_POINT ( 'NONE', #6884 ) ;
#4533=CARTESIAN_POINT ( 'NONE',  ( 34.51370081393729095, 101.0775402828204363, 15.68973407569667877 ) ) ;
#4550=DIRECTION ( 'NONE',  ( 0.000000000000000000, 0.000000000000000000, -1.000000000000000000 ) ) ;
#4553=ADVANCED_FACE ( 'NONE', ( #14734 ), #7651, .T. ) ;
#4559=CARTESIAN_POINT ( 'NONE',  ( -31.47058823529412663, 102.2673069760056421, 11.00000000000000000 ) ) ;
#4569=CARTESIAN_POINT ( 'NONE',  ( 32.35455048062397054, 95.67796756487049947, 15.49337032400452863 ) ) ;
#4570=CIRCLE ( 'NONE', #6725, 75.00000000000001421 ) ;
#4573=CARTESIAN_POINT ( 'NONE',  ( -12.24154204929785550, 106.2975094407664329, 16.61985167119452811 ) ) ;
#4577=DIRECTION ( 'NONE',  ( 0.000000000000000000, 0.000000000000000000, 1.000000000000000000 ) ) ;
#4578=VERTEX_POINT ( 'NONE', #2042 ) ;
#4588=CARTESIAN_POINT ( 'NONE',  ( 12.39897948556635754, 100.2360479454198696, -16.00000000000000000 ) ) ;
#4592=VECTOR ( 'NONE', #3070, 1000.000000000000000 ) ;
#4595=ORIENTED_EDGE ( 'NONE', *, *, #14240, .T. ) ;
#4599=LINE ( 'NONE', #3378, #14948 ) ;
#4603=CARTESIAN_POINT ( 'NONE',  ( 29.70588235294119173, 96.53269163155674448, 10.99999999999999645 ) ) ;
#4608=CARTESIAN_POINT ( 'NONE',  ( 12.39897948556635576, 73.96800191783272282, 16.00000000000000000 ) ) ;
#4610=CARTESIAN_POINT ( 'NONE',  ( -25.00000000000000000, 81.24038404635962252, 31.00000000000000000 ) ) ;
#4629=DIRECTION ( 'NONE',  ( -0.000000000000000000, -0.000000000000000000, 1.000000000000000000 ) ) ;
#4647=CARTESIAN_POINT ( 'NONE',  ( -8.076099607191862262, 62.48290387921809952, 20.00000000000000000 ) ) ;
#4648=CARTESIAN_POINT ( 'NONE',  ( 0.000000000000000000, 0.000000000000000000, -23.50000000000000000 ) ) ;
#4649=CARTESIAN_POINT ( 'NONE',  ( -10.54368182729039738, 106.4795995572428353, 18.98024639174783701 ) ) ;
#4666=DIRECTION ( 'NONE',  ( -0.000000000000000000, -0.000000000000000000, 1.000000000000000000 ) ) ;
#4686=DIRECTION ( 'NONE',  ( 1.000000000000000000, 0.000000000000000000, 0.000000000000000000 ) ) ;
#4689=ORIENTED_EDGE ( 'NONE', *, *, #11282, .F. ) ;
#4690=CARTESIAN_POINT ( 'NONE',  ( 22.05882352941176094, 71.68269180561141241, 23.50000000000000355 ) ) ;
#4696=DIRECTION ( 'NONE',  ( 0.000000000000000000, 1.000000000000000000, 0.000000000000000000 ) ) ;
#4701=VERTEX_POINT ( 'NONE', #1362 ) ;
#4705=FACE_OUTER_BOUND ( 'NONE', #8778, .T. ) ;
#4711=DIRECTION ( 'NONE',  ( -0.000000000000000000, -0.000000000000000000, -1.000000000000000000 ) ) ;
#4716=CIRCLE ( 'NONE', #12225, 4.999999999999995559 ) ;
#4722=CARTESIAN_POINT ( 'NONE',  ( 29.70588235294119173, 96.53269163155674448, 10.99999999999999645 ) ) ;
#4730=VECTOR ( 'NONE', #5599, 1000.000000000000000 ) ;
#4732=DIRECTION ( 'NONE',  ( 0.000000000000000000, 0.000000000000000000, -1.000000000000000000 ) ) ;
#4736=ORIENTED_EDGE ( 'NONE', *, *, #8888, .F. ) ;
#4739=AXIS2_PLACEMENT_3D ( 'NONE', #1684, #10944, #1762 ) ;
#4744=EDGE_LOOP ( 'NONE', ( #7598, #7600, #10772, #14208 ) ) ;
#4746=ORIENTED_EDGE ( 'NONE', *, *, #1797, .T. ) ;
#4750=DIRECTION ( 'NONE',  ( -1.000000000000000000, 0.000000000000000000, 0.000000000000000000 ) ) ;
#4755=CARTESIAN_POINT ( 'NONE',  ( 25.00000000000000000, 81.24038404635960831, 31.00000000000000000 ) ) ;
#4761=CARTESIAN_POINT ( 'NONE',  ( 7.500000000000000000, 106.7368258849775202, 20.00000000000000355 ) ) ;
#4762=DIRECTION ( 'NONE',  ( 0.000000000000000000, 0.000000000000000000, -1.000000000000000000 ) ) ;
#4763=DIRECTION ( 'NONE',  ( 0.000000000000000000, 0.000000000000000000, 1.000000000000000000 ) ) ;
#4767=CARTESIAN_POINT ( 'NONE',  ( -9.707422895060656032, 94.50306011459642264, 19.49540453443646726 ) ) ;
#4783=DIRECTION ( 'NONE',  ( 0.2941176470588238723, -0.9557692240748189016, 0.000000000000000000 ) ) ;
#4800=EDGE_CURVE ( 'NONE', #721, #3540, #858, .T. ) ;
#4805=EDGE_CURVE ( 'NONE', #7414, #3127, #9076, .T. ) ;
#4808=ORIENTED_EDGE ( 'NONE', *, *, #13914, .T. ) ;
#4809=EDGE_CURVE ( 'NONE', #10105, #4879, #10534, .T. ) ;
#4826=CARTESIAN_POINT ( 'NONE',  ( 12.37198577373457198, 106.2823362334109447, 16.13593661559556480 ) ) ;
#4830=EDGE_LOOP ( 'NONE', ( #12384, #11292 ) ) ;
#4832=VERTEX_POINT ( 'NONE', #14485 ) ;
#4833=EDGE_LOOP ( 'NONE', ( #12494, #12287, #13338, #9823, #3834, #3375, #3509, #819, #12361 ) ) ;
#4837=CARTESIAN_POINT ( 'NONE',  ( 35.00000000000000000, 81.24038404635960831, -23.50000000000000000 ) ) ;
#4839=VERTEX_POINT ( 'NONE', #8473 ) ;
#4842=CIRCLE ( 'NONE', #13826, 101.0000000000000284 ) ;
#4848=DIRECTION ( 'NONE',  ( 0.000000000000000000, 0.000000000000000000, -1.000000000000000000 ) ) ;
#4850=CARTESIAN_POINT ( 'NONE',  ( -12.39897948556635754, 73.96800191783273704, -16.00000000000000000 ) ) ;
#4856=ORIENTED_EDGE ( 'NONE', *, *, #10490, .T. ) ;
#4863=ORIENTED_EDGE ( 'NONE', *, *, #9991, .F. ) ;
#4869=CARTESIAN_POINT ( 'NONE',  ( -12.39897948556635754, 94.18739463280904545, -16.00000000000000000 ) ) ;
#4870=CIRCLE ( 'NONE', #12617, 22.00000000000001421 ) ;
#4872=PLANE ( 'NONE',  #11424 ) ;
#4875=CARTESIAN_POINT ( 'NONE',  ( -12.39897948556635754, 100.2360479454198696, 16.00000000000000000 ) ) ;
#4879=VERTEX_POINT ( 'NONE', #7839 ) ;
#4885=DIRECTION ( 'NONE',  ( -0.000000000000000000, -0.000000000000000000, -1.000000000000000000 ) ) ;
#4893=CARTESIAN_POINT ( 'NONE',  ( -22.05882352941176450, 71.68269180561142662, -23.50000000000000000 ) ) ;
#4895=AXIS2_PLACEMENT_3D ( 'NONE', #7485, #8930, #6342 ) ;
#4902=CARTESIAN_POINT ( 'NONE',  ( 34.44830544488820578, 94.94374256356070418, 16.00000000000000000 ) ) ;
#4910=CARTESIAN_POINT ( 'NONE',  ( 12.46748823216054092, 106.2711901036690705, 15.65608700630148675 ) ) ;
#4912=EDGE_CURVE ( 'NONE', #508, #2772, #4976, .T. ) ;
#4916=CARTESIAN_POINT ( 'NONE',  ( 18.52941176470587692, 60.21346111671358159, 16.00000000000000000 ) ) ;
#4917=ORIENTED_EDGE ( 'NONE', *, *, #12475, .F. ) ;
#4918=CIRCLE ( 'NONE', #801, 10.00000000000000355 ) ;
#4920=ADVANCED_FACE ( 'NONE', ( #14404 ), #4012, .F. ) ;
#4922=CARTESIAN_POINT ( 'NONE',  ( 7.500000000000000000, 59.24038404635959409, 15.00000000000000000 ) ) ;
#4931=CARTESIAN_POINT ( 'NONE',  ( -7.500000000000000888, 59.24038404635959409, -15.00000000000000000 ) ) ;
#4932=CARTESIAN_POINT ( 'NONE',  ( 5.204748896376250896E-15, 85.00000000000000000, 46.00000000000000000 ) ) ;
#4933=CARTESIAN_POINT ( 'NONE',  ( 0.000000000000000000, 0.000000000000000000, -26.00000000000000000 ) ) ;
#4937=CARTESIAN_POINT ( 'NONE',  ( 47.00000000000001421, 81.24038404635960831, 26.00000000000000000 ) ) ;
#4942=ORIENTED_EDGE ( 'NONE', *, *, #15022, .T. ) ;
#4953=CIRCLE ( 'NONE', #2524, 22.00000000000000355 ) ;
#4965=AXIS2_PLACEMENT_3D ( 'NONE', #13807, #3401, #13965 ) ;
#4968=ORIENTED_EDGE ( 'NONE', *, *, #8110, .T. ) ;
#4972=CARTESIAN_POINT ( 'NONE',  ( -31.62605012285503392, 102.2189371620064691, -12.30800327571618347 ) ) ;
#4976=CIRCLE ( 'NONE', #11270, 22.00000000000000000 ) ;
#4982=DIRECTION ( 'NONE',  ( 1.000000000000000000, 0.000000000000000000, 0.000000000000000000 ) ) ;
#4987=DIRECTION ( 'NONE',  ( 0.000000000000000000, 0.000000000000000000, 1.000000000000000000 ) ) ;
#4992=CARTESIAN_POINT ( 'NONE',  ( -22.05882352941176450, 71.68269180561142662, 13.50000000000000533 ) ) ;
#4995=VECTOR ( 'NONE', #3781, 1000.000000000000000 ) ;
#5024=FACE_OUTER_BOUND ( 'NONE', #739, .T. ) ;
#5030=CARTESIAN_POINT ( 'NONE',  ( -11.26445476358325237, 106.4056658731563942, -18.30680964731275040 ) ) ;
#5038=DIRECTION ( 'NONE',  ( -0.000000000000000000, -0.000000000000000000, 1.000000000000000000 ) ) ;
#5041=CARTESIAN_POINT ( 'NONE',  ( -8.915162460657663601, 94.58113943660329426, 19.80393736615727462 ) ) ;
#5045=DIRECTION ( 'NONE',  ( -0.000000000000000000, -1.000000000000000000, -0.000000000000000000 ) ) ;
#5053=CARTESIAN_POINT ( 'NONE',  ( 12.07377633196514211, 61.83297368684233675, -17.10072941380095202 ) ) ;
#5062=VERTEX_POINT ( 'NONE', #5642 ) ;
#5072=CARTESIAN_POINT ( 'NONE',  ( -4.999999999999996447, 85.00000000000000000, 46.00000000000000000 ) ) ;
#5074=ORIENTED_EDGE ( 'NONE', *, *, #5337, .T. ) ;
#5079=CARTESIAN_POINT ( 'NONE',  ( -29.73684948645749415, 96.52317830260923870, 11.65681975620353938 ) ) ;
#5081=DIRECTION ( 'NONE',  ( 0.000000000000000000, 0.000000000000000000, -1.000000000000000000 ) ) ;
#5085=CARTESIAN_POINT ( 'NONE',  ( 7.500000000000007105, 85.00000000000000000, 31.00000000000000000 ) ) ;
#5108=AXIS2_PLACEMENT_3D ( 'NONE', #296, #6125, #10768 ) ;
#5111=CARTESIAN_POINT ( 'NONE',  ( -31.47058823529411242, 102.2673069760056421, -11.33188329630078606 ) ) ;
#5118=DIRECTION ( 'NONE',  ( 0.9557692240748190127, -0.2941176470588235392, 6.631981242474902501E-16 ) ) ;
#5120=FACE_OUTER_BOUND ( 'NONE', #5751, .T. ) ;
#5126=ORIENTED_EDGE ( 'NONE', *, *, #2182, .T. ) ;
#5128=CARTESIAN_POINT ( 'NONE',  ( -8.635299310232698033, 74.50321615228340022, 19.90320263233616771 ) ) ;
#5134=CARTESIAN_POINT ( 'NONE',  ( -30.33578517098776217, 96.33676874097989185, -13.50363573142180584 ) ) ;
#5148=CARTESIAN_POINT ( 'NONE',  ( -25.00000000000000000, 81.24038404635962252, -26.00000000000000000 ) ) ;
#5165=DIRECTION ( 'NONE',  ( 0.000000000000000000, 0.000000000000000000, -1.000000000000000000 ) ) ;
#5180=VECTOR ( 'NONE', #11483, 1000.000000000000000 ) ;
#5183=ORIENTED_EDGE ( 'NONE', *, *, #13412, .F. ) ;
#5184=LINE ( 'NONE', #4055, #5692 ) ;
#5186=FACE_OUTER_BOUND ( 'NONE', #13858, .T. ) ;
#5188=EDGE_CURVE ( 'NONE', #7196, #1809, #1397, .T. ) ;
#5201=ORIENTED_EDGE ( 'NONE', *, *, #11920, .T. ) ;
#5203=VERTEX_POINT ( 'NONE', #13080 ) ;
#5207=CARTESIAN_POINT ( 'NONE',  ( 12.39897948556635399, 61.76783392443435616, -16.00000000000000000 ) ) ;
#5210=CARTESIAN_POINT ( 'NONE',  ( -30.68146655995339245, 96.22723358344983069, -14.04702900388066311 ) ) ;
#5224=ORIENTED_EDGE ( 'NONE', *, *, #9173, .F. ) ;
#5226=LINE ( 'NONE', #8697, #13687 ) ;
#5237=ORIENTED_EDGE ( 'NONE', *, *, #1854, .F. ) ;
#5244=DIRECTION ( 'NONE',  ( -0.000000000000000000, -0.000000000000000000, -1.000000000000000000 ) ) ;
#5251=CARTESIAN_POINT ( 'NONE',  ( 17.27884612037405887, 39.14960378788569528, 11.00000000000000000 ) ) ;
#5252=CARTESIAN_POINT ( 'NONE',  ( -18.52941176470586981, 60.21346111671361001, -26.00000000000000000 ) ) ;
#5259=FACE_OUTER_BOUND ( 'NONE', #7509, .T. ) ;
#5260=VERTEX_POINT ( 'NONE', #13237 ) ;
#5264=CARTESIAN_POINT ( 'NONE',  ( -35.50766591049261223, 100.5715065882092745, -15.96896126722779208 ) ) ;
#5267=CARTESIAN_POINT ( 'NONE',  ( -12.05137958362237960, 94.23255994477487718, 17.08976535968791310 ) ) ;
#5269=VERTEX_POINT ( 'NONE', #3126 ) ;
#5303=ORIENTED_EDGE ( 'NONE', *, *, #7034, .T. ) ;
#5316=EDGE_CURVE ( 'NONE', #4479, #6344, #342, .T. ) ;
#5321=CARTESIAN_POINT ( 'NONE',  ( 33.83210567914650824, 95.16559600367021687, -15.96768719852781615 ) ) ;
#5326=ADVANCED_FACE ( 'NONE', ( #7821 ), #13200, .T. ) ;
#5329=CARTESIAN_POINT ( 'NONE',  ( 0.000000000000000000, 0.000000000000000000, -31.00000000000000000 ) ) ;
#5337=EDGE_CURVE ( 'NONE', #11614, #1920, #6520, .T. ) ;
#5343=DIRECTION ( 'NONE',  ( -0.000000000000000000, 1.000000000000000000, -0.000000000000000000 ) ) ;
#5347=STYLED_ITEM ( 'NONE', ( #6720 ), #2938 ) ;
#5358=VERTEX_POINT ( 'NONE', #4279 ) ;
#5364=CARTESIAN_POINT ( 'NONE',  ( 11.10542050108867507, 94.34972528831985983, 18.51161449521946167 ) ) ;
#5374=EDGE_CURVE ( 'NONE', #337, #3540, #2279, .T. ) ;
#5391=CARTESIAN_POINT ( 'NONE',  ( -29.70588235294118107, 96.53269163155674448, 10.99999999999999645 ) ) ;
#5396=DIRECTION ( 'NONE',  ( 0.000000000000000000, 0.000000000000000000, -1.000000000000000000 ) ) ;
#5399=ORIENTED_EDGE ( 'NONE', *, *, #4416, .T. ) ;
#5403=AXIS2_PLACEMENT_3D ( 'NONE', #1227, #11636, #9121 ) ;
#5406=DIRECTION ( 'NONE',  ( 0.000000000000000000, 0.000000000000000000, -1.000000000000000000 ) ) ;
#5408=CARTESIAN_POINT ( 'NONE',  ( -12.28299834225913223, 61.79111542428977799, 16.56818924177463614 ) ) ;
#5421=VERTEX_POINT ( 'NONE', #7970 ) ;
#5426=ORIENTED_EDGE ( 'NONE', *, *, #10637, .T. ) ;
#5442=LINE ( 'NONE', #8846, #10319 ) ;
#5443=CARTESIAN_POINT ( 'NONE',  ( 25.00000000000000000, 81.24038404635960831, 31.00000000000000000 ) ) ;
#5452=DIRECTION ( 'NONE',  ( -0.000000000000000000, 0.000000000000000000, 1.000000000000000000 ) ) ;
#5460=AXIS2_PLACEMENT_3D ( 'NONE', #10905, #5566, #13197 ) ;
#5461=EDGE_CURVE ( 'NONE', #2447, #7811, #12723, .T. ) ;
#5482=CARTESIAN_POINT ( 'NONE',  ( 33.23060097332286489, 95.37689352056796110, -15.83317473434553335 ) ) ;
#5484=ORIENTED_EDGE ( 'NONE', *, *, #1125, .T. ) ;
#5486=CARTESIAN_POINT ( 'NONE',  ( -12.39897948556635754, 61.76783392443436327, 16.00000000000000000 ) ) ;
#5492=CARTESIAN_POINT ( 'NONE',  ( -9.448652591187071792, 74.40292581525912397, -19.61336856585178623 ) ) ;
#5496=CARTESIAN_POINT ( 'NONE',  ( 11.08614924580848360, 94.35111528408442894, -18.49588680517285511 ) ) ;
#5507=CARTESIAN_POINT ( 'NONE',  ( 9.714076971208447375, 106.5585699559772621, -19.49498877141799014 ) ) ;
#5509=VERTEX_POINT ( 'NONE', #3733 ) ;
#5516=DIRECTION ( 'NONE',  ( -0.2941176470588237613, -0.9557692240748189016, 0.000000000000000000 ) ) ;
#5518=ADVANCED_FACE ( 'NONE', ( #11934 ), #13685, .T. ) ;
#5522=CARTESIAN_POINT ( 'NONE',  ( -12.50000000000000000, 100.2235002382176248, 15.00000000000000000 ) ) ;
#5528=CARTESIAN_POINT ( 'NONE',  ( -36.08010649850015028, 100.2464683348682684, 16.00000000000000000 ) ) ;
#5536=CARTESIAN_POINT ( 'NONE',  ( -12.39897948556635754, 100.2360479454198696, 16.00000000000000000 ) ) ;
#5539=CARTESIAN_POINT ( 'NONE',  ( -31.47058823529412663, 102.2673069760056563, -10.99999999999999645 ) ) ;
#5561=FILL_AREA_STYLE_COLOUR ( '', #6574 ) ;
#5566=DIRECTION ( 'NONE',  ( -0.000000000000000000, -0.000000000000000000, 1.000000000000000000 ) ) ;
#5569=CARTESIAN_POINT ( 'NONE',  ( 17.27884612037405887, 39.14960378788569528, 16.00000000000000000 ) ) ;
#5574=LINE ( 'NONE', #9062, #6866 ) ;
#5584=VERTEX_POINT ( 'NONE', #11853 ) ;
#5592=DIRECTION ( 'NONE',  ( -0.000000000000000000, -0.000000000000000000, 1.000000000000000000 ) ) ;
#5597=ORIENTED_EDGE ( 'NONE', *, *, #7115, .F. ) ;
#5598=AXIS2_PLACEMENT_3D ( 'NONE', #5909, #12828, #2417 ) ;
#5599=DIRECTION ( 'NONE',  ( 0.000000000000000000, 0.000000000000000000, -1.000000000000000000 ) ) ;
#5601=CIRCLE ( 'NONE', #11435, 4.999999999999995559 ) ;
#5602=ORIENTED_EDGE ( 'NONE', *, *, #4800, .T. ) ;
#5611=CARTESIAN_POINT ( 'NONE',  ( 12.50000000000000000, 106.2673515243510991, -15.00000000000000355 ) ) ;
#5615=ORIENTED_EDGE ( 'NONE', *, *, #6947, .T. ) ;
#5618=CARTESIAN_POINT ( 'NONE',  ( -27.94117647058823550, 90.79807628710781842, 16.00000000000000000 ) ) ;
#5623=DIRECTION ( 'NONE',  ( -0.000000000000000000, -0.000000000000000000, 1.000000000000000000 ) ) ;
#5631=FACE_OUTER_BOUND ( 'NONE', #2627, .T. ) ;
#5633=( NAMED_UNIT ( * ) PLANE_ANGLE_UNIT ( ) SI_UNIT ( $, .RADIAN. ) );
#5642=CARTESIAN_POINT ( 'NONE',  ( -12.39897948556635754, 61.76783392443436327, -16.00000000000000000 ) ) ;
#5665=VERTEX_POINT ( 'NONE', #52 ) ;
#5667=FACE_OUTER_BOUND ( 'NONE', #4744, .T. ) ;
#5668=CARTESIAN_POINT ( 'NONE',  ( 7.500000000000000000, 61.74746958378133144, 20.00000000000000000 ) ) ;
#5673=EDGE_LOOP ( 'NONE', ( #1426, #4595, #1858, #1868 ) ) ;
#5678=ORIENTED_EDGE ( 'NONE', *, *, #5374, .T. ) ;
#5679=ORIENTED_EDGE ( 'NONE', *, *, #10951, .F. ) ;
#5689=ORIENTED_EDGE ( 'NONE', *, *, #4180, .T. ) ;
#5692=VECTOR ( 'NONE', #2898, 1000.000000000000000 ) ;
#5695=EDGE_CURVE ( 'NONE', #5665, #1689, #13212, .T. ) ;
#5698=EDGE_CURVE ( 'NONE', #13514, #14649, #10310, .T. ) ;
#5702=ORIENTED_EDGE ( 'NONE', *, *, #6638, .T. ) ;
#5708=EDGE_CURVE ( 'NONE', #1445, #13430, #11526, .T. ) ;
#5715=CARTESIAN_POINT ( 'NONE',  ( 7.787692492290230639, 94.68070094645281642, -20.00000000000000355 ) ) ;
#5716=DIRECTION ( 'NONE',  ( -0.000000000000000000, -0.000000000000000000, 1.000000000000000000 ) ) ;
#5730=VERTEX_POINT ( 'NONE', #14177 ) ;
#5732=CARTESIAN_POINT ( 'NONE',  ( -7.500000000000000888, 62.55197838597913318, -20.00000000000000000 ) ) ;
#5738=ORIENTED_EDGE ( 'NONE', *, *, #10712, .T. ) ;
#5742=DIRECTION ( 'NONE',  ( -0.000000000000000000, -0.000000000000000000, 1.000000000000000000 ) ) ;
#5747=ORIENTED_EDGE ( 'NONE', *, *, #7773, .F. ) ;
#5751=EDGE_LOOP ( 'NONE', ( #13791, #5303, #609, #6112 ) ) ;
#5757=CARTESIAN_POINT ( 'NONE',  ( 5.204748896376250896E-15, 85.00000000000000000, 46.00000000000000000 ) ) ;
#5761=DIRECTION ( 'NONE',  ( -1.000000000000000000, 0.000000000000000000, 0.000000000000000000 ) ) ;
#5771=CARTESIAN_POINT ( 'NONE',  ( -34.44830544488820578, 94.94374256356071839, 16.00000000000000000 ) ) ;
#5773=CARTESIAN_POINT ( 'NONE',  ( 0.000000000000000000, 0.000000000000000000, -16.00000000000000000 ) ) ;
#5775=CARTESIAN_POINT ( 'NONE',  ( 5.204748896376250896E-15, 85.00000000000000000, 31.00000000000000000 ) ) ;
#5793=CARTESIAN_POINT ( 'NONE',  ( -11.47656068366043236, 61.94660012053729048, -18.08543280684388677 ) ) ;
#5798=CIRCLE ( 'NONE', #1209, 5.000000000000001776 ) ;
#5801=DIRECTION ( 'NONE',  ( 1.000000000000000000, 0.000000000000000000, 0.000000000000000000 ) ) ;
#5804=CARTESIAN_POINT ( 'NONE',  ( 0.000000000000000000, 0.000000000000000000, -31.00000000000000000 ) ) ;
#5811=AXIS2_PLACEMENT_3D ( 'NONE', #7809, #4035, #8646 ) ;
#5817=EDGE_LOOP ( 'NONE', ( #7340, #5834, #9517, #11870, #8013 ) ) ;
#5825=CIRCLE ( 'NONE', #7766, 63.00000000000000000 ) ;
#5826=DIRECTION ( 'NONE',  ( -1.000000000000000000, 0.000000000000000000, 0.000000000000000000 ) ) ;
#5828=DIRECTION ( 'NONE',  ( 1.000000000000000000, 0.000000000000000000, 0.000000000000000000 ) ) ;
#5829=DIRECTION ( 'NONE',  ( -0.000000000000000000, -0.000000000000000000, -1.000000000000000000 ) ) ;
#5834=ORIENTED_EDGE ( 'NONE', *, *, #7365, .T. ) ;
#5856=CARTESIAN_POINT ( 'NONE',  ( -10.80358476664834910, 106.4534462909512769, -18.76728514983857465 ) ) ;
#5863=CARTESIAN_POINT ( 'NONE',  ( 0.000000000000000000, 0.000000000000000000, -31.00000000000000000 ) ) ;
#5866=CARTESIAN_POINT ( 'NONE',  ( -22.05882352941176450, 71.68269180561142662, 16.00000000000000000 ) ) ;
#5867=DIRECTION ( 'NONE',  ( 0.000000000000000000, 0.000000000000000000, 1.000000000000000000 ) ) ;
#5872=CARTESIAN_POINT ( 'NONE',  ( -34.44830544488820578, 94.94374256356073261, -16.00000000000000000 ) ) ;
#5891=FACE_OUTER_BOUND ( 'NONE', #4833, .T. ) ;
#5892=CIRCLE ( 'NONE', #9045, 17.00000000000000000 ) ;
#5898=VERTEX_POINT ( 'NONE', #13182 ) ;
#5908=ORIENTED_EDGE ( 'NONE', *, *, #2182, .F. ) ;
#5909=CARTESIAN_POINT ( 'NONE',  ( 5.204748896376250896E-15, 85.00000000000000000, 46.00000000000000000 ) ) ;
#5923=CARTESIAN_POINT ( 'NONE',  ( -9.714076971208447375, 106.5585699559772479, 19.49498877141798658 ) ) ;
#5924=DIRECTION ( 'NONE',  ( -1.000000000000000000, 0.000000000000000000, 0.000000000000000000 ) ) ;
#5931=EDGE_CURVE ( 'NONE', #9955, #1777, #2305, .T. ) ;
#5935=DIRECTION ( 'NONE',  ( 0.000000000000000000, 0.000000000000000000, 1.000000000000000000 ) ) ;
#5940=CARTESIAN_POINT ( 'NONE',  ( 12.50000000000000000, 100.2235002382176248, 15.00000000000000000 ) ) ;
#5947=VERTEX_POINT ( 'NONE', #6181 ) ;
#5958=CARTESIAN_POINT ( 'NONE',  ( 47.00000000000001421, 81.24038404635960831, -16.00000000000000000 ) ) ;
#5963=ADVANCED_FACE ( 'NONE', ( #14389 ), #13103, .F. ) ;
#5977=CARTESIAN_POINT ( 'NONE',  ( -7.500000000000000888, 74.62405778299650194, 20.00000000000000000 ) ) ;
#5989=CARTESIAN_POINT ( 'NONE',  ( 25.00000000000000000, 81.24038404635960831, 23.50000000000000355 ) ) ;
#5999=CARTESIAN_POINT ( 'NONE',  ( 5.204748896376250896E-15, 85.00000000000000000, 46.00000000000000000 ) ) ;
#6003=DIRECTION ( 'NONE',  ( 1.000000000000000000, 0.000000000000000000, 0.000000000000000000 ) ) ;
#6008=ORIENTED_EDGE ( 'NONE', *, *, #3021, .F. ) ;
#6018=EDGE_CURVE ( 'NONE', #143, #13983, #11289, .T. ) ;
#6019=LINE ( 'NONE', #9590, #4194 ) ;
#6026=CARTESIAN_POINT ( 'NONE',  ( -29.95643228365058164, 96.45524571768991962, -12.60642518152332237 ) ) ;
#6028=ORIENTED_EDGE ( 'NONE', *, *, #1988, .T. ) ;
#6041=CIRCLE ( 'NONE', #7989, 107.0000000000000284 ) ;
#6042=CARTESIAN_POINT ( 'NONE',  ( -12.39897948556635754, 61.76783392443436327, 16.00000000000000000 ) ) ;
#6048=B_SPLINE_CURVE_WITH_KNOTS ( 'NONE', 3,
 ( #641, #11755, #14528, #5267, #4131, #13387, #10813, #2986, #7610, #10527, #127, #4767, #7382, #5041, #14027, #8243, #14298, #3908 ),
 .UNSPECIFIED., .F., .F.,
 ( 4, 2, 2, 2, 2, 2, 2, 2, 4 ),
 ( 0.001002887730653555286, 0.001856445934617267663, 0.002710004138580980257, 0.003563562342544692417, 0.004417120546508405445, 0.005270678750472117605, 0.006124236954435829765, 0.006977795158399542792, 0.007831353362363254952 ),
 .UNSPECIFIED. ) ;
#6053=CIRCLE ( 'NONE', #9216, 17.00000000000000000 ) ;
#6058=ORIENTED_EDGE ( 'NONE', *, *, #6282, .T. ) ;
#6064=CIRCLE ( 'NONE', #14576, 95.00000000000001421 ) ;
#6070=AXIS2_PLACEMENT_3D ( 'NONE', #12295, #8606, #14242 ) ;
#6075=CARTESIAN_POINT ( 'NONE',  ( -7.829984960685305140, 106.7136390683879910, -20.00000000000000000 ) ) ;
#6078=CARTESIAN_POINT ( 'NONE',  ( 0.000000000000000000, 0.000000000000000000, 16.00000000000000000 ) ) ;
#6079=AXIS2_PLACEMENT_3D ( 'NONE', #4610, #4762, #8316 ) ;
#6084=ORIENTED_EDGE ( 'NONE', *, *, #1535, .T. ) ;
#6091=ADVANCED_FACE ( 'NONE', ( #11279 ), #3226, .T. ) ;
#6097=DIRECTION ( 'NONE',  ( 1.000000000000000000, 0.000000000000000000, 0.000000000000000000 ) ) ;
#6108=CARTESIAN_POINT ( 'NONE',  ( 11.62509980388830222, 61.91833518448028428, -17.84018927347701577 ) ) ;
#6112=ORIENTED_EDGE ( 'NONE', *, *, #2272, .F. ) ;
#6115=ORIENTED_EDGE ( 'NONE', *, *, #8514, .F. ) ;
#6121=DIRECTION ( 'NONE',  ( -1.000000000000000000, 0.000000000000000000, 0.000000000000000000 ) ) ;
#6125=DIRECTION ( 'NONE',  ( 0.000000000000000000, 0.000000000000000000, 1.000000000000000000 ) ) ;
#6140=DIRECTION ( 'NONE',  ( -0.000000000000000000, -0.000000000000000000, 1.000000000000000000 ) ) ;
#6141=DIRECTION ( 'NONE',  ( -0.000000000000000000, -0.000000000000000000, -1.000000000000000000 ) ) ;
#6149=AXIS2_PLACEMENT_3D ( 'NONE', #9726, #8594, #14455 ) ;
#6159=VERTEX_POINT ( 'NONE', #12789 ) ;
#6162=CARTESIAN_POINT ( 'NONE',  ( 12.50000000000000000, 100.2235002382176248, 15.33678752976415716 ) ) ;
#6169=AXIS2_PLACEMENT_3D ( 'NONE', #2637, #1506, #6121 ) ;
#6173=CYLINDRICAL_SURFACE ( 'NONE', #11290, 22.00000000000001421 ) ;
#6176=ADVANCED_FACE ( 'NONE', ( #10281 ), #9285, .T. ) ;
#6177=ORIENTED_EDGE ( 'NONE', *, *, #3021, .T. ) ;
#6178=DIRECTION ( 'NONE',  ( -0.000000000000000000, -0.000000000000000000, 1.000000000000000000 ) ) ;
#6179=AXIS2_PLACEMENT_3D ( 'NONE', #698, #1982, #11252 ) ;
#6181=CARTESIAN_POINT ( 'NONE',  ( -18.52941176470586981, 60.21346111671361001, -16.00000000000000000 ) ) ;
#6183=CARTESIAN_POINT ( 'NONE',  ( 10.87743925404099876, 62.05426862177564118, -18.69798886497097712 ) ) ;
#6191=CARTESIAN_POINT ( 'NONE',  ( 12.50000000000000000, 100.2235002382176248, -15.00000000000000000 ) ) ;
#6192=ORIENTED_EDGE ( 'NONE', *, *, #6798, .F. ) ;
#6227=CARTESIAN_POINT ( 'NONE',  ( 12.39897948556635754, 100.2360479454198696, 16.00000000000000000 ) ) ;
#6231=CARTESIAN_POINT ( 'NONE',  ( -29.70588235294118107, 96.53269163155674448, -10.99999999999999645 ) ) ;
#6232=EDGE_CURVE ( 'NONE', #14105, #7249, #2452, .T. ) ;
#6233=CARTESIAN_POINT ( 'NONE',  ( -32.45630819848046400, 101.9391205390361534, -14.06872601623944519 ) ) ;
#6240=CARTESIAN_POINT ( 'NONE',  ( -4.999999999999996447, 85.00000000000000000, 31.00000000000000000 ) ) ;
#6248=LINE ( 'NONE', #1642, #820 ) ;
#6258=DIRECTION ( 'NONE',  ( -1.000000000000000000, 0.000000000000000000, 0.000000000000000000 ) ) ;
#6262=EDGE_CURVE ( 'NONE', #2264, #1542, #6992, .T. ) ;
#6269=ORIENTED_EDGE ( 'NONE', *, *, #3139, .F. ) ;
#6273=CARTESIAN_POINT ( 'NONE',  ( -30.33882973767906321, 96.33581297378611907, 13.50942224097978617 ) ) ;
#6275=CIRCLE ( 'NONE', #9668, 22.00000000000000000 ) ;
#6276=CARTESIAN_POINT ( 'NONE',  ( 32.10455955028198360, 102.0624585623582306, -13.51511155787191854 ) ) ;
#6279=CARTESIAN_POINT ( 'NONE',  ( 42.00000000000000711, 81.24038404635960831, 26.00000000000000000 ) ) ;
#6282=EDGE_CURVE ( 'NONE', #944, #7811, #3678, .T. ) ;
#6297=VECTOR ( 'NONE', #6514, 1000.000000000000000 ) ;
#6299=LINE ( 'NONE', #9803, #6841 ) ;
#6300=CARTESIAN_POINT ( 'NONE',  ( -34.09969740539978034, 101.2725728942521215, -15.50446122302711949 ) ) ;
#6304=EDGE_LOOP ( 'NONE', ( #7195, #1679, #12345, #5126, #3107 ) ) ;
#6308=AXIS2_PLACEMENT_3D ( 'NONE', #7567, #14264, #376 ) ;
#6325=DIRECTION ( 'NONE',  ( 0.000000000000000000, 1.000000000000000000, 0.000000000000000000 ) ) ;
#6327=AXIS2_PLACEMENT_3D ( 'NONE', #13846, #9347, #9489 ) ;
#6342=DIRECTION ( 'NONE',  ( -1.000000000000000000, 0.000000000000000000, -0.000000000000000000 ) ) ;
#6344=VERTEX_POINT ( 'NONE', #4893 ) ;
#6345=DIRECTION ( 'NONE',  ( 0.000000000000000000, 0.000000000000000000, 1.000000000000000000 ) ) ;
#6354=EDGE_CURVE ( 'NONE', #7414, #7196, #3647, .T. ) ;
#6358=DIRECTION ( 'NONE',  ( 0.000000000000000000, 0.000000000000000000, -1.000000000000000000 ) ) ;
#6361=CARTESIAN_POINT ( 'NONE',  ( 0.000000000000000000, 0.000000000000000000, 16.00000000000000000 ) ) ;
#6367=CYLINDRICAL_SURFACE ( 'NONE', #6179, 63.00000000000000000 ) ;
#6382=CARTESIAN_POINT ( 'NONE',  ( -34.93865171984689511, 100.8681255216228578, -15.83776386865433672 ) ) ;
#6388=FACE_OUTER_BOUND ( 'NONE', #3807, .T. ) ;
#6389=UNCERTAINTY_MEASURE_WITH_UNIT (LENGTH_MEASURE( 1.000000000000000082E-05 ), #675, 'distance_accuracy_value', 'NONE');
#6392=CIRCLE ( 'NONE', #7376, 22.00000000000000000 ) ;
#6393=ORIENTED_EDGE ( 'NONE', *, *, #3854, .T. ) ;
#6396=DIRECTION ( 'NONE',  ( 0.000000000000000000, 1.000000000000000000, -0.000000000000000000 ) ) ;
#6430=DIRECTION ( 'NONE',  ( 0.9557692240748186796, 0.2941176470588241498, 0.000000000000000000 ) ) ;
#6433=LINE ( 'NONE', #14498, #627 ) ;
#6483=CARTESIAN_POINT ( 'NONE',  ( 10.21436410913239889, 94.45034564433045432, 19.23824501837256307 ) ) ;
#6487=ORIENTED_EDGE ( 'NONE', *, *, #9477, .T. ) ;
#6494=CARTESIAN_POINT ( 'NONE',  ( -32.65070903206048314, 101.8685403450051723, 14.31792419690431473 ) ) ;
#6496=DIRECTION ( 'NONE',  ( -0.2941176470588241498, 0.9557692240748186796, 0.000000000000000000 ) ) ;
#6498=EDGE_LOOP ( 'NONE', ( #6766, #14233, #4005, #13216, #13407, #2387, #9622, #5678 ) ) ;
#6501=EDGE_CURVE ( 'NONE', #11614, #1392, #9930, .T. ) ;
#6512=DIRECTION ( 'NONE',  ( 0.000000000000000000, -0.000000000000000000, -1.000000000000000000 ) ) ;
#6514=DIRECTION ( 'NONE',  ( 0.000000000000000000, 0.000000000000000000, -1.000000000000000000 ) ) ;
#6516=CARTESIAN_POINT ( 'NONE',  ( 29.73684948645749415, 96.52317830260923870, -11.65681975620353406 ) ) ;
#6519=ORIENTED_EDGE ( 'NONE', *, *, #5695, .T. ) ;
#6520=LINE ( 'NONE', #6598, #2769 ) ;
#6524=DIRECTION ( 'NONE',  ( 0.000000000000000000, 0.000000000000000000, -1.000000000000000000 ) ) ;
#6525=AXIS2_PLACEMENT_3D ( 'NONE', #6995, #10430, #4750 ) ;
#6535=ORIENTED_EDGE ( 'NONE', *, *, #7034, .F. ) ;
#6536=CARTESIAN_POINT ( 'NONE',  ( 11.10403672352021331, 74.17481381252333961, -18.51301757891052091 ) ) ;
#6537=CARTESIAN_POINT ( 'NONE',  ( 25.00000000000000000, 81.24038404635960831, 31.00000000000000000 ) ) ;
#6553=VECTOR ( 'NONE', #5742, 1000.000000000000000 ) ;
#6558=CARTESIAN_POINT ( 'NONE',  ( -19.99999999999998224, 64.99230723708768664, 26.00000000000000000 ) ) ;
#6559=CARTESIAN_POINT ( 'NONE',  ( 34.93865171984692353, 100.8681255216228436, 15.83776386865434382 ) ) ;
#6564=AXIS2_PLACEMENT_3D ( 'NONE', #10506, #5867, #11517 ) ;
#6566=ORIENTED_EDGE ( 'NONE', *, *, #9964, .F. ) ;
#6574=COLOUR_RGB ( '', 0.31764706, 0.68627451, 0.89019608) ;
#6575=DIRECTION ( 'NONE',  ( 0.000000000000000000, 1.000000000000000000, -0.000000000000000000 ) ) ;
#6587=DIRECTION ( 'NONE',  ( -1.000000000000000000, 0.000000000000000000, 0.000000000000000000 ) ) ;
#6593=AXIS2_PLACEMENT_3D ( 'NONE', #2222, #12697, #1092 ) ;
#6595=CARTESIAN_POINT ( 'NONE',  ( 33.38013186279886924, 95.32466787866007962, -15.87266497586409209 ) ) ;
#6598=CARTESIAN_POINT ( 'NONE',  ( -7.499999999999996447, 85.00000000000000000, 46.00000000000000000 ) ) ;
#6601=CIRCLE ( 'NONE', #9281, 4.999999999999995559 ) ;
#6608=CARTESIAN_POINT ( 'NONE',  ( -12.50000000000000000, 106.2673515243510991, -15.00000000000000000 ) ) ;
#6620=CARTESIAN_POINT ( 'NONE',  ( -25.00000000000000000, 81.24038404635962252, -26.00000000000000000 ) ) ;
#6636=CARTESIAN_POINT ( 'NONE',  ( 31.95875033779849872, 102.1112180006092984, 13.22918226575834311 ) ) ;
#6638=EDGE_CURVE ( 'NONE', #8983, #8663, #10265, .T. ) ;
#6643=EDGE_LOOP ( 'NONE', ( #12363, #11650, #7639, #11707, #2245 ) ) ;
#6644=AXIS2_PLACEMENT_3D ( 'NONE', #14873, #9312, #7946 ) ;
#6645=CARTESIAN_POINT ( 'NONE',  ( -12.50000000000000000, 100.2235002382176248, -15.00000000000000000 ) ) ;
#6653=VERTEX_POINT ( 'NONE', #8134 ) ;
#6655=EDGE_CURVE ( 'NONE', #7623, #2264, #8103, .T. ) ;
#6675=DIRECTION ( 'NONE',  ( -0.000000000000000000, -0.000000000000000000, 1.000000000000000000 ) ) ;
#6677=AXIS2_PLACEMENT_3D ( 'NONE', #13139, #14049, #12992 ) ;
#6684=DIRECTION ( 'NONE',  ( -1.000000000000000000, 0.000000000000000000, 0.000000000000000000 ) ) ;
#6689=CARTESIAN_POINT ( 'NONE',  ( -10.88080562889580705, 74.20685544768620900, -18.69467976711750978 ) ) ;
#6692=DIRECTION ( 'NONE',  ( -1.000000000000000000, 0.000000000000000000, 0.000000000000000000 ) ) ;
#6697=ORIENTED_EDGE ( 'NONE', *, *, #2089, .F. ) ;
#6702=CARTESIAN_POINT ( 'NONE',  ( 0.000000000000000000, 0.000000000000000000, 20.00000000000000000 ) ) ;
#6705=CARTESIAN_POINT ( 'NONE',  ( 9.260566377415146988, 106.5986160369160558, -19.68264575353697055 ) ) ;
#6710=CARTESIAN_POINT ( 'NONE',  ( -12.28299983316191302, 61.79111512501306436, -16.56818193787248816 ) ) ;
#6711=CARTESIAN_POINT ( 'NONE',  ( 31.47058823529414440, 102.2673069760056421, 11.33188329630078783 ) ) ;
#6713=VERTEX_POINT ( 'NONE', #5085 ) ;
#6720=PRESENTATION_STYLE_ASSIGNMENT (( #10376 ) ) ;
#6723=ORIENTED_EDGE ( 'NONE', *, *, #7949, .T. ) ;
#6725=AXIS2_PLACEMENT_3D ( 'NONE', #11758, #1423, #11686 ) ;
#6730=CARTESIAN_POINT ( 'NONE',  ( 29.70588235294119173, 96.53269163155674448, -79.80561291909842225 ) ) ;
#6751=CARTESIAN_POINT ( 'NONE',  ( -12.49999999999999645, 106.2673515243510849, 15.33085973118639167 ) ) ;
#6752=FACE_OUTER_BOUND ( 'NONE', #13558, .T. ) ;
#6754=CARTESIAN_POINT ( 'NONE',  ( -12.34196858416779996, 73.97755844198597686, -16.27929523640516862 ) ) ;
#6766=ORIENTED_EDGE ( 'NONE', *, *, #4800, .F. ) ;
#6770=CARTESIAN_POINT ( 'NONE',  ( 8.791121401460923579, 106.6383652286472881, -19.83320147728688454 ) ) ;
#6772=ORIENTED_EDGE ( 'NONE', *, *, #3017, .T. ) ;
#6779=CARTESIAN_POINT ( 'NONE',  ( 8.635722793752535154, 94.60824746434937538, 19.90313979694426649 ) ) ;
#6784=AXIS2_PLACEMENT_3D ( 'NONE', #4107, #1678, #7363 ) ;
#6787=CARTESIAN_POINT ( 'NONE',  ( 8.914534555419061590, 74.46880876796768689, 19.80411369943039901 ) ) ;
#6798=EDGE_CURVE ( 'NONE', #11834, #259, #2929, .T. ) ;
#6800=ADVANCED_FACE ( 'NONE', ( #8358 ), #4872, .T. ) ;
#6805=VERTEX_POINT ( 'NONE', #8279 ) ;
#6806=AXIS2_PLACEMENT_3D ( 'NONE', #3697, #15013, #12956 ) ;
#6823=B_SPLINE_CURVE_WITH_KNOTS ( 'NONE', 3,
 ( #2161, #13486, #6779, #11363, #6483, #5364, #815, #897, #962, #9069 ),
 .UNSPECIFIED., .F., .F.,
 ( 4, 2, 2, 2, 4 ),
 ( 0.000000000000000000, 0.001708674401391109023, 0.003417348802782218045, 0.005126023204173327068, 0.006834697605564436090 ),
 .UNSPECIFIED. ) ;
#6827=EDGE_LOOP ( 'NONE', ( #7641, #10385, #3701, #5237 ) ) ;
#6832=B_SPLINE_CURVE_WITH_KNOTS ( 'NONE', 3,
 ( #5207, #11057, #5053, #6108, #495, #14311, #6183, #350, #3923, #12116, #8538, #14245, #658, #4148 ),
 .UNSPECIFIED., .F., .F.,
 ( 4, 2, 2, 2, 2, 2, 4 ),
 ( 0.000000000000000000, 0.001716022237784524482, 0.002574033356676786941, 0.003432044475569049399, 0.004290055594461312724, 0.005148066713353574748, 0.006864088951138102267 ),
 .UNSPECIFIED. ) ;
#6833=CARTESIAN_POINT ( 'NONE',  ( -7.500000000000000888, 62.55197838597913318, 20.00000000000000000 ) ) ;
#6841=VECTOR ( 'NONE', #8667, 1000.000000000000000 ) ;
#6853=CARTESIAN_POINT ( 'NONE',  ( -12.50000000000000000, 61.74746958378133144, 15.00000000000000000 ) ) ;
#6854=ADVANCED_FACE ( 'NONE', ( #11538 ), #12659, .F. ) ;
#6856=DIRECTION ( 'NONE',  ( 0.000000000000000000, 0.000000000000000000, -1.000000000000000000 ) ) ;
#6861=LINE ( 'NONE', #1182, #2053 ) ;
#6866=VECTOR ( 'NONE', #2380, 1000.000000000000000 ) ;
#6871=FACE_OUTER_BOUND ( 'NONE', #10546, .T. ) ;
#6878=ORIENTED_EDGE ( 'NONE', *, *, #3525, .F. ) ;
#6884=CARTESIAN_POINT ( 'NONE',  ( -22.05882352941176450, 71.68269180561142662, 23.50000000000000355 ) ) ;
#6897=ORIENTED_EDGE ( 'NONE', *, *, #7210, .F. ) ;
#6910=CARTESIAN_POINT ( 'NONE',  ( -10.87743925404099699, 62.05426862177564118, 18.69798886497097357 ) ) ;
#6916=AXIS2_PLACEMENT_3D ( 'NONE', #6558, #9904, #11212 ) ;
#6919=ORIENTED_EDGE ( 'NONE', *, *, #530, .F. ) ;
#6924=EDGE_LOOP ( 'NONE', ( #10173, #5484, #10064, #10441 ) ) ;
#6927=CARTESIAN_POINT ( 'NONE',  ( -25.00000000000000000, 81.24038404635962252, -31.00000000000000000 ) ) ;
#6942=B_SPLINE_CURVE_WITH_KNOTS ( 'NONE', 3,
 ( #13426, #13500, #4251, #2036, #754, #9847, #3104, #13566, #11309, #3031, #6494, #2948, #10998, #10003, #8866, #14729, #831, #911, #7717, #5528 ),
 .UNSPECIFIED., .F., .F.,
 ( 4, 2, 2, 2, 2, 2, 2, 2, 2, 4 ),
 ( 0.000000000000000000, 0.0009815662899613972463, 0.001472349434942093376, 0.001963132579922789289, 0.002944698869884177211, 0.003926265159845564699, 0.004907831449806952621, 0.005889397739768340544, 0.006870964029729727598, 0.007852530319691115521 ),
 .UNSPECIFIED. ) ;
#6945=CARTESIAN_POINT ( 'NONE',  ( -25.00000000000000000, 81.24038404635962252, 26.00000000000000000 ) ) ;
#6947=EDGE_CURVE ( 'NONE', #13983, #14637, #1052, .T. ) ;
#6974=CARTESIAN_POINT ( 'NONE',  ( 29.95643228365060295, 96.45524571768993383, 12.60642518152332769 ) ) ;
#6978=CARTESIAN_POINT ( 'NONE',  ( 22.05882352941176094, 71.68269180561141241, 13.50000000000000533 ) ) ;
#6980=FACE_OUTER_BOUND ( 'NONE', #14173, .T. ) ;
#6992=LINE ( 'NONE', #6853, #13828 ) ;
#6994=VECTOR ( 'NONE', #3817, 1000.000000000000000 ) ;
#6995=CARTESIAN_POINT ( 'NONE',  ( 0.000000000000000000, 0.000000000000000000, 23.50000000000000355 ) ) ;
#6999=CARTESIAN_POINT ( 'NONE',  ( -9.717538815323484513, 62.24844358264333266, -19.51802576651051879 ) ) ;
#7002=DIRECTION ( 'NONE',  ( 0.2941176470588238168, -0.9557692240748187906, 0.000000000000000000 ) ) ;
#7034=EDGE_CURVE ( 'NONE', #12827, #1689, #9375, .T. ) ;
#7056=PRODUCT_CONTEXT ( 'NONE', #674, 'mechanical' ) ;
#7058=MECHANICAL_DESIGN_GEOMETRIC_PRESENTATION_REPRESENTATION('',(#11202),#529);
#7063=FACE_OUTER_BOUND ( 'NONE', #2115, .T. ) ;
#7065=ORIENTED_EDGE ( 'NONE', *, *, #73, .T. ) ;
#7068=EDGE_LOOP ( 'NONE', ( #10474, #1866, #6566, #1086 ) ) ;
#7087=ADVANCED_FACE ( 'NONE', ( #122 ), #14166, .T. ) ;
#7095=ORIENTED_EDGE ( 'NONE', *, *, #12158, .T. ) ;
#7097=CARTESIAN_POINT ( 'NONE',  ( 0.000000000000000000, 0.000000000000000000, -16.00000000000000000 ) ) ;
#7107=CARTESIAN_POINT ( 'NONE',  ( -25.00000000000000000, 81.24038404635962252, -23.50000000000000000 ) ) ;
#7115=EDGE_CURVE ( 'NONE', #3630, #9614, #10695, .T. ) ;
#7121=ORIENTED_EDGE ( 'NONE', *, *, #10237, .F. ) ;
#7125=ORIENTED_EDGE ( 'NONE', *, *, #266, .T. ) ;
#7129=FACE_OUTER_BOUND ( 'NONE', #4492, .T. ) ;
#7133=CIRCLE ( 'NONE', #4496, 63.00000000000000000 ) ;
#7136=ADVANCED_FACE ( 'NONE', ( #7625 ), #4165, .T. ) ;
#7142=CIRCLE ( 'NONE', #3772, 5.000000000000001776 ) ;
#7147=VERTEX_POINT ( 'NONE', #9826 ) ;
#7148=DIRECTION ( 'NONE',  ( -1.000000000000000000, 0.000000000000000000, 0.000000000000000000 ) ) ;
#7157=ORIENTED_EDGE ( 'NONE', *, *, #10151, .T. ) ;
#7161=CARTESIAN_POINT ( 'NONE',  ( 0.000000000000000000, 0.000000000000000000, -16.00000000000000000 ) ) ;
#7168=CARTESIAN_POINT ( 'NONE',  ( 18.52941176470587692, 60.21346111671358159, -26.00000000000000000 ) ) ;
#7174=ORIENTED_EDGE ( 'NONE', *, *, #2677, .T. ) ;
#7179=VECTOR ( 'NONE', #13563, 1000.000000000000000 ) ;
#7184=AXIS2_PLACEMENT_3D ( 'NONE', #2145, #14987, #12782 ) ;
#7191=CARTESIAN_POINT ( 'NONE',  ( -11.08463629228402603, 74.17659209477393745, -18.49742775384897442 ) ) ;
#7195=ORIENTED_EDGE ( 'NONE', *, *, #6354, .T. ) ;
#7196=VERTEX_POINT ( 'NONE', #3001 ) ;
#7199=EDGE_LOOP ( 'NONE', ( #14968, #12518, #5399, #8127 ) ) ;
#7210=EDGE_CURVE ( 'NONE', #4832, #6805, #6832, .T. ) ;
#7215=AXIS2_PLACEMENT_3D ( 'NONE', #5251, #11612, #15020 ) ;
#7220=ORIENTED_EDGE ( 'NONE', *, *, #6947, .F. ) ;
#7231=ORIENTED_EDGE ( 'NONE', *, *, #12801, .F. ) ;
#7235=CARTESIAN_POINT ( 'NONE',  ( 9.115592515563379905, 106.6114291000284027, 19.74294316973679386 ) ) ;
#7238=EDGE_CURVE ( 'NONE', #331, #10950, #9704, .T. ) ;
#7239=CARTESIAN_POINT ( 'NONE',  ( -30.18932686484984629, 96.38267619380719964, -13.21651853314490488 ) ) ;
#7241=ORIENTED_EDGE ( 'NONE', *, *, #11969, .T. ) ;
#7246=FACE_OUTER_BOUND ( 'NONE', #3342, .T. ) ;
#7247=CARTESIAN_POINT ( 'NONE',  ( 12.50000000000000000, 100.2235002382176248, -15.33678752976415716 ) ) ;
#7249=VERTEX_POINT ( 'NONE', #7544 ) ;
#7259=EDGE_CURVE ( 'NONE', #331, #14939, #1576, .T. ) ;
#7263=CYLINDRICAL_SURFACE ( 'NONE', #13089, 10.00000000000000178 ) ;
#7275=CARTESIAN_POINT ( 'NONE',  ( 35.79340317121621240, 100.4136097276748387, -16.00000000000000355 ) ) ;
#7280=DIRECTION ( 'NONE',  ( 0.000000000000000000, 0.000000000000000000, -1.000000000000000000 ) ) ;
#7295=VECTOR ( 'NONE', #2528, 1000.000000000000000 ) ;
#7302=DIRECTION ( 'NONE',  ( 0.000000000000000000, 0.000000000000000000, 1.000000000000000000 ) ) ;
#7306=EDGE_CURVE ( 'NONE', #1809, #5203, #7847, .T. ) ;
#7308=DIRECTION ( 'NONE',  ( 0.2941176470588241498, 0.9557692240748186796, 0.000000000000000000 ) ) ;
#7336=FACE_OUTER_BOUND ( 'NONE', #245, .T. ) ;
#7338=DIRECTION ( 'NONE',  ( 1.000000000000000000, 0.000000000000000000, 0.000000000000000000 ) ) ;
#7340=ORIENTED_EDGE ( 'NONE', *, *, #14984, .T. ) ;
#7343=DIRECTION ( 'NONE',  ( -0.000000000000000000, -0.000000000000000000, 1.000000000000000000 ) ) ;
#7346=TOROIDAL_SURFACE ( 'NONE', #2500, 102.0000000000000142, 5.000000000000000000 ) ;
#7347=ORIENTED_EDGE ( 'NONE', *, *, #6501, .T. ) ;
#7356=CARTESIAN_POINT ( 'NONE',  ( -12.50000000000000000, 59.24038404635959409, 20.00000000000000000 ) ) ;
#7363=DIRECTION ( 'NONE',  ( 1.000000000000000000, 0.000000000000000000, 0.000000000000000000 ) ) ;
#7365=EDGE_CURVE ( 'NONE', #27, #5421, #9448, .T. ) ;
#7368=DIRECTION ( 'NONE',  ( -1.000000000000000000, 0.000000000000000000, 0.000000000000000000 ) ) ;
#7369=EDGE_CURVE ( 'NONE', #14085, #1445, #3645, .T. ) ;
#7376=AXIS2_PLACEMENT_3D ( 'NONE', #12212, #7645, #14722 ) ;
#7380=CARTESIAN_POINT ( 'NONE',  ( -33.83495342806088502, 101.3902949203996116, -15.35262818605210988 ) ) ;
#7382=CARTESIAN_POINT ( 'NONE',  ( -9.449524216731115089, 94.52924706620449058, 19.61300924954587188 ) ) ;
#7392=CARTESIAN_POINT ( 'NONE',  ( -31.47058823529412663, 102.2673069760056563, -79.80561291909842225 ) ) ;
#7394=AXIS2_PLACEMENT_3D ( 'NONE', #6078, #1316, #7368 ) ;
#7398=ORIENTED_EDGE ( 'NONE', *, *, #4047, .F. ) ;
#7400=ADVANCED_FACE ( 'NONE', ( #253 ), #105, .F. ) ;
#7404=CARTESIAN_POINT ( 'NONE',  ( -32.35455048062396344, 95.67796756487054211, -15.49337032400452507 ) ) ;
#7414=VERTEX_POINT ( 'NONE', #3537 ) ;
#7424=CARTESIAN_POINT ( 'NONE',  ( 25.00000000000000000, 81.24038404635960831, 13.50000000000000533 ) ) ;
#7431=CARTESIAN_POINT ( 'NONE',  ( 31.63177518854776338, 102.2170822241992596, -12.29884221335728967 ) ) ;
#7449=LINE ( 'NONE', #1625, #14360 ) ;
#7457=PLANE ( 'NONE',  #10586 ) ;
#7458=DIRECTION ( 'NONE',  ( 0.000000000000000000, 0.000000000000000000, -1.000000000000000000 ) ) ;
#7459=DIRECTION ( 'NONE',  ( -1.000000000000000000, 0.000000000000000000, 0.000000000000000000 ) ) ;
#7461=B_SPLINE_CURVE_WITH_KNOTS ( 'NONE', 3,
 ( #5732, #2320, #2160, #6999, #2097, #1042, #5793, #13869, #6710, #9217 ),
 .UNSPECIFIED., .F., .F.,
 ( 4, 2, 2, 2, 4 ),
 ( 0.000000000000000000, 0.001715760189696190381, 0.003431520379392380762, 0.005147280569088571144, 0.006863040758784761525 ),
 .UNSPECIFIED. ) ;
#7469=FACE_OUTER_BOUND ( 'NONE', #5817, .T. ) ;
#7475=DIRECTION ( 'NONE',  ( -1.000000000000000000, 0.000000000000000000, 0.000000000000000000 ) ) ;
#7485=CARTESIAN_POINT ( 'NONE',  ( 12.50000000000000000, 40.62019202317980415, -16.00000000000000000 ) ) ;
#7486=ORIENTED_EDGE ( 'NONE', *, *, #10994, .F. ) ;
#7509=EDGE_LOOP ( 'NONE', ( #3849, #10163, #8158, #4240, #8349 ) ) ;
#7510=CARTESIAN_POINT ( 'NONE',  ( 30.33882973767905966, 96.33581297378609065, -13.50942224097978261 ) ) ;
#7524=DIRECTION ( 'NONE',  ( 1.000000000000000000, 0.000000000000000000, 0.000000000000000000 ) ) ;
#7544=CARTESIAN_POINT ( 'NONE',  ( 35.00000000000000000, 81.24038404635960831, 23.50000000000000355 ) ) ;
#7567=CARTESIAN_POINT ( 'NONE',  ( -7.500000000000000888, 59.24038404635959409, 15.00000000000000000 ) ) ;
#7575=CARTESIAN_POINT ( 'NONE',  ( 0.000000000000000000, 0.000000000000000000, -20.00000000000000000 ) ) ;
#7579=AXIS2_PLACEMENT_3D ( 'NONE', #14643, #5452, #13344 ) ;
#7590=EDGE_CURVE ( 'NONE', #11955, #14956, #3596, .T. ) ;
#7595=CARTESIAN_POINT ( 'NONE',  ( 29.70588235294118462, 96.53269163155671606, -11.33021639467929731 ) ) ;
#7598=ORIENTED_EDGE ( 'NONE', *, *, #13487, .T. ) ;
#7600=ORIENTED_EDGE ( 'NONE', *, *, #6262, .T. ) ;
#7610=CARTESIAN_POINT ( 'NONE',  ( -10.88232432232081770, 94.37491168429329491, 18.69329470938989957 ) ) ;
#7613=DIRECTION ( 'NONE',  ( 0.000000000000000000, 0.000000000000000000, -1.000000000000000000 ) ) ;
#7614=AXIS2_PLACEMENT_3D ( 'NONE', #8622, #1647, #1799 ) ;
#7623=VERTEX_POINT ( 'NONE', #10873 ) ;
#7625=FACE_OUTER_BOUND ( 'NONE', #8174, .T. ) ;
#7628=ORIENTED_EDGE ( 'NONE', *, *, #10648, .T. ) ;
#7630=EDGE_CURVE ( 'NONE', #5584, #11834, #6053, .T. ) ;
#7636=CARTESIAN_POINT ( 'NONE',  ( 31.71893208106492423, 102.1896529572239558, 12.62523369519216665 ) ) ;
#7638=CARTESIAN_POINT ( 'NONE',  ( 25.00000000000000000, 81.24038404635960831, 23.50000000000000355 ) ) ;
#7639=ORIENTED_EDGE ( 'NONE', *, *, #4180, .F. ) ;
#7641=ORIENTED_EDGE ( 'NONE', *, *, #7369, .T. ) ;
#7645=DIRECTION ( 'NONE',  ( -0.000000000000000000, -0.000000000000000000, 1.000000000000000000 ) ) ;
#7651=TOROIDAL_SURFACE ( 'NONE', #11556, 17.00000000000001066, 5.000000000000000000 ) ;
#7653=FACE_OUTER_BOUND ( 'NONE', #13806, .T. ) ;
#7660=CARTESIAN_POINT ( 'NONE',  ( -29.86020745210522875, 96.48508785265609333, 12.30285360678859696 ) ) ;
#7690=DIRECTION ( 'NONE',  ( -0.000000000000000000, 0.000000000000000000, 1.000000000000000000 ) ) ;
#7695=LINE ( 'NONE', #13542, #3193 ) ;
#7703=ORIENTED_EDGE ( 'NONE', *, *, #1294, .T. ) ;
#7704=ORIENTED_EDGE ( 'NONE', *, *, #3287, .F. ) ;
#7708=EDGE_LOOP ( 'NONE', ( #9912, #1041, #12748, #7174, #3018, #12625, #6008, #1644 ) ) ;
#7713=( NAMED_UNIT ( * ) SI_UNIT ( $, .STERADIAN. ) SOLID_ANGLE_UNIT ( ) );
#7717=CARTESIAN_POINT ( 'NONE',  ( -35.79340317121619819, 100.4136097276748103, 16.00000000000000000 ) ) ;
#7718=ORIENTED_EDGE ( 'NONE', *, *, #6232, .F. ) ;
#7721=ORIENTED_EDGE ( 'NONE', *, *, #9655, .F. ) ;
#7722=DIRECTION ( 'NONE',  ( 1.000000000000000000, 0.000000000000000000, 0.000000000000000000 ) ) ;
#7723=EDGE_CURVE ( 'NONE', #11013, #5269, #13463, .T. ) ;
#7726=LINE ( 'NONE', #12373, #10663 ) ;
#7736=LINE ( 'NONE', #4837, #5180 ) ;
#7744=DIRECTION ( 'NONE',  ( -1.000000000000000000, 0.000000000000000000, 0.000000000000000000 ) ) ;
#7745=AXIS2_PLACEMENT_3D ( 'NONE', #2894, #330, #1765 ) ;
#7751=VECTOR ( 'NONE', #12097, 1000.000000000000000 ) ;
#7754=VECTOR ( 'NONE', #1162, 1000.000000000000000 ) ;
#7757=SURFACE_STYLE_USAGE ( .BOTH. , #12400 ) ;
#7760=CARTESIAN_POINT ( 'NONE',  ( 11.92530613726453659, 94.24865542230074311, -17.34466199971670264 ) ) ;
#7761=AXIS2_PLACEMENT_3D ( 'NONE', #5989, #11575, #1159 ) ;
#7766=AXIS2_PLACEMENT_3D ( 'NONE', #4933, #4848, #2493 ) ;
#7773=EDGE_CURVE ( 'NONE', #944, #1495, #12111, .T. ) ;
#7774=AXIS2_PLACEMENT_3D ( 'NONE', #14660, #12452, #13579 ) ;
#7779=ORIENTED_EDGE ( 'NONE', *, *, #13043, .T. ) ;
#7781=ORIENTED_EDGE ( 'NONE', *, *, #978, .F. ) ;
#7785=CARTESIAN_POINT ( 'NONE',  ( 33.08820577230234505, 101.7009610928536887, 14.78158739605038896 ) ) ;
#7800=CARTESIAN_POINT ( 'NONE',  ( 0.000000000000000000, 0.000000000000000000, -20.00000000000000000 ) ) ;
#7809=CARTESIAN_POINT ( 'NONE',  ( 0.000000000000000000, 0.000000000000000000, 16.00000000000000000 ) ) ;
#7811=VERTEX_POINT ( 'NONE', #1388 ) ;
#7815=CARTESIAN_POINT ( 'NONE',  ( 0.000000000000000000, 0.000000000000000000, 20.00000000000000000 ) ) ;
#7817=ADVANCED_FACE ( 'NONE', ( #9192 ), #3589, .F. ) ;
#7819=CARTESIAN_POINT ( 'NONE',  ( 7.500000000000000000, 94.70348462437907244, 20.00000000000000000 ) ) ;
#7821=FACE_OUTER_BOUND ( 'NONE', #12009, .T. ) ;
#7826=CARTESIAN_POINT ( 'NONE',  ( -11.10542050108867329, 94.34972528831985983, -18.51161449521946523 ) ) ;
#7830=FACE_OUTER_BOUND ( 'NONE', #1197, .T. ) ;
#7832=FILL_AREA_STYLE ('',( #5561 ) ) ;
#7833=ORIENTED_EDGE ( 'NONE', *, *, #3691, .T. ) ;
#7834=ADVANCED_FACE ( 'NONE', ( #6980 ), #4110, .T. ) ;
#7836=CARTESIAN_POINT ( 'NONE',  ( 9.707422895060663137, 94.50306011459642264, -19.49540453443647436 ) ) ;
#7839=CARTESIAN_POINT ( 'NONE',  ( -27.94117647058823550, 90.79807628710781842, -16.00000000000000000 ) ) ;
#7844=CARTESIAN_POINT ( 'NONE',  ( -12.50000000000000000, 59.24038404635959409, 20.00000000000000000 ) ) ;
#7847=LINE ( 'NONE', #7927, #2665 ) ;
#7851=AXIS2_PLACEMENT_3D ( 'NONE', #4294, #7690, #798 ) ;
#7865=FACE_OUTER_BOUND ( 'NONE', #12094, .T. ) ;
#7869=( NAMED_UNIT ( * ) SI_UNIT ( $, .STERADIAN. ) SOLID_ANGLE_UNIT ( ) );
#7905=CARTESIAN_POINT ( 'NONE',  ( -11.46932393819253626, 106.3836852522821346, 18.05815993169795064 ) ) ;
#7910=FACE_OUTER_BOUND ( 'NONE', #11043, .T. ) ;
#7915=CARTESIAN_POINT ( 'NONE',  ( -25.00000000000000000, 81.24038404635962252, -16.00000000000000000 ) ) ;
#7920=CARTESIAN_POINT ( 'NONE',  ( 42.00000000000000711, 81.24038404635960831, 31.00000000000000000 ) ) ;
#7927=CARTESIAN_POINT ( 'NONE',  ( 31.47058823529413729, 102.2673069760056563, -79.80561291909842225 ) ) ;
#7939=CARTESIAN_POINT ( 'NONE',  ( 11.92448918074846986, 74.04612619069749258, 17.34622847719485605 ) ) ;
#7943=DIRECTION ( 'NONE',  ( 0.000000000000000000, 1.000000000000000000, -0.000000000000000000 ) ) ;
#7945=ORIENTED_EDGE ( 'NONE', *, *, #5188, .F. ) ;
#7946=DIRECTION ( 'NONE',  ( -1.000000000000000000, 0.000000000000000000, 0.000000000000000000 ) ) ;
#7949=EDGE_CURVE ( 'NONE', #10570, #13797, #2817, .T. ) ;
#7970=CARTESIAN_POINT ( 'NONE',  ( 27.94117647058824616, 90.79807628710781842, 23.50000000000000355 ) ) ;
#7981=LINE ( 'NONE', #1099, #3077 ) ;
#7984=VERTEX_POINT ( 'NONE', #14214 ) ;
#7989=AXIS2_PLACEMENT_3D ( 'NONE', #11164, #5396, #6587 ) ;
#8002=DIRECTION ( 'NONE',  ( -0.2941176470588238168, 0.9557692240748187906, -0.000000000000000000 ) ) ;
#8012=AXIS2_PLACEMENT_3D ( 'NONE', #6361, #11946, #1533 ) ;
#8013=ORIENTED_EDGE ( 'NONE', *, *, #4407, .T. ) ;
#8024=ORIENTED_EDGE ( 'NONE', *, *, #8420, .T. ) ;
#8027=CARTESIAN_POINT ( 'NONE',  ( -27.94117647058823550, 90.79807628710781842, 23.50000000000000355 ) ) ;
#8036=LINE ( 'NONE', #12593, #9471 ) ;
#8075=DIRECTION ( 'NONE',  ( -0.000000000000000000, -0.000000000000000000, 1.000000000000000000 ) ) ;
#8083=LINE ( 'NONE', #4603, #2731 ) ;
#8088=CARTESIAN_POINT ( 'NONE',  ( 7.500000000000000000, 74.62405778299650194, 20.00000000000000000 ) ) ;
#8090=CYLINDRICAL_SURFACE ( 'NONE', #3483, 107.0000000000000284 ) ;
#8103=B_SPLINE_CURVE_WITH_KNOTS ( 'NONE', 3,
 ( #11494, #12838, #12696, #11713, #1305, #1226, #3355, #5923, #9408, #4649, #9269, #3285, #7905, #2362, #13921, #4573, #1091, #2138, #6751, #10339 ),
 .UNSPECIFIED., .F., .F.,
 ( 4, 2, 2, 2, 2, 2, 2, 2, 2, 4 ),
 ( 8.673617379884035472E-19, 0.0009783702772842232508, 0.001467555415926338454, 0.001956740554568453874, 0.002935110831852691653, 0.003913481109136930300, 0.004891851386421167645, 0.005870221663705405858, 0.006848591940989644071, 0.007826962218273881416 ),
 .UNSPECIFIED. ) ;
#8110=EDGE_CURVE ( 'NONE', #7623, #7147, #6041, .T. ) ;
#8116=ADVANCED_FACE ( 'NONE', ( #4268 ), #9438, .T. ) ;
#8121=AXIS2_PLACEMENT_3D ( 'NONE', #6537, #714, #13611 ) ;
#8127=ORIENTED_EDGE ( 'NONE', *, *, #2736, .T. ) ;
#8129=CARTESIAN_POINT ( 'NONE',  ( 30.68146655995342087, 96.22723358344990174, 14.04702900388066844 ) ) ;
#8131=CARTESIAN_POINT ( 'NONE',  ( -9.703618315745389467, 62.24871376222712627, 19.49715125027359974 ) ) ;
#8134=CARTESIAN_POINT ( 'NONE',  ( 31.47058823529413374, 102.2673069760056563, 26.00000000000000000 ) ) ;
#8143=DIRECTION ( 'NONE',  ( -0.000000000000000000, 1.000000000000000000, -0.000000000000000000 ) ) ;
#8148=ORIENTED_EDGE ( 'NONE', *, *, #5461, .T. ) ;
#8158=ORIENTED_EDGE ( 'NONE', *, *, #3691, .F. ) ;
#8172=VERTEX_POINT ( 'NONE', #3420 ) ;
#8174=EDGE_LOOP ( 'NONE', ( #9381, #2261, #9691, #1803 ) ) ;
#8182=ORIENTED_EDGE ( 'NONE', *, *, #10699, .T. ) ;
#8188=ORIENTED_EDGE ( 'NONE', *, *, #3543, .F. ) ;
#8189=CARTESIAN_POINT ( 'NONE',  ( -8.914534555419061590, 74.46880876796768689, -19.80411369943039901 ) ) ;
#8200=CARTESIAN_POINT ( 'NONE',  ( 30.33578517098777638, 96.33676874097987763, 13.50363573142180940 ) ) ;
#8204=CARTESIAN_POINT ( 'NONE',  ( 0.000000000000000000, 0.000000000000000000, -16.00000000000000000 ) ) ;
#8208=DIRECTION ( 'NONE',  ( -0.000000000000000000, 1.000000000000000000, -0.000000000000000000 ) ) ;
#8210=CARTESIAN_POINT ( 'NONE',  ( -7.500000000000000888, 106.7368258849775202, -20.00000000000000000 ) ) ;
#8217=EDGE_CURVE ( 'NONE', #9064, #14934, #3150, .T. ) ;
#8234=EDGE_CURVE ( 'NONE', #5947, #11955, #6275, .T. ) ;
#8241=VECTOR ( 'NONE', #4666, 1000.000000000000000 ) ;
#8243=CARTESIAN_POINT ( 'NONE',  ( -8.072481656125564342, 94.65682832148054615, 19.97535367358595693 ) ) ;
#8258=DIRECTION ( 'NONE',  ( -0.000000000000000000, -0.000000000000000000, -1.000000000000000000 ) ) ;
#8264=CARTESIAN_POINT ( 'NONE',  ( -11.92448918074847342, 74.04612619069749258, -17.34622847719484540 ) ) ;
#8267=ORIENTED_EDGE ( 'NONE', *, *, #382, .T. ) ;
#8279=CARTESIAN_POINT ( 'NONE',  ( 7.500000000000000888, 62.55197838597913318, -20.00000000000000000 ) ) ;
#8295=DIRECTION ( 'NONE',  ( -0.000000000000000000, -0.000000000000000000, 1.000000000000000000 ) ) ;
#8308=FACE_OUTER_BOUND ( 'NONE', #6643, .T. ) ;
#8313=VECTOR ( 'NONE', #10375, 1000.000000000000000 ) ;
#8315=DIRECTION ( 'NONE',  ( 0.000000000000000000, 0.000000000000000000, 1.000000000000000000 ) ) ;
#8316=DIRECTION ( 'NONE',  ( 1.000000000000000000, 0.000000000000000000, 0.000000000000000000 ) ) ;
#8324=CYLINDRICAL_SURFACE ( 'NONE', #2619, 5.000000000000000888 ) ;
#8330=ORIENTED_EDGE ( 'NONE', *, *, #13396, .T. ) ;
#8336=ADVANCED_FACE ( 'NONE', ( #1438 ), #7263, .F. ) ;
#8344=ORIENTED_EDGE ( 'NONE', *, *, #13441, .T. ) ;
#8349=ORIENTED_EDGE ( 'NONE', *, *, #921, .F. ) ;
#8355=CARTESIAN_POINT ( 'NONE',  ( 31.59365702568383938, 102.2290646705776282, -12.13969626787233835 ) ) ;
#8358=FACE_OUTER_BOUND ( 'NONE', #1030, .T. ) ;
#8366=CARTESIAN_POINT ( 'NONE',  ( -12.18091848848563430, 106.3044177073317087, -16.76518324937863014 ) ) ;
#8380=CIRCLE ( 'NONE', #6677, 75.00000000000001421 ) ;
#8381=CARTESIAN_POINT ( 'NONE',  ( -32.10716661655236948, 102.0615849490104949, -13.52016324361725275 ) ) ;
#8387=VECTOR ( 'NONE', #14235, 1000.000000000000000 ) ;
#8389=VERTEX_POINT ( 'NONE', #4937 ) ;
#8399=CARTESIAN_POINT ( 'NONE',  ( -29.70588235294118107, 96.53269163155674448, -10.99999999999999645 ) ) ;
#8404=VERTEX_POINT ( 'NONE', #11775 ) ;
#8420=EDGE_CURVE ( 'NONE', #12827, #7196, #10411, .T. ) ;
#8424=ORIENTED_EDGE ( 'NONE', *, *, #12801, .T. ) ;
#8427=EDGE_CURVE ( 'NONE', #9614, #3630, #5798, .T. ) ;
#8439=CARTESIAN_POINT ( 'NONE',  ( -7.500000000000000000, 74.62405778299650194, -20.00000000000000000 ) ) ;
#8441=DIRECTION ( 'NONE',  ( -0.000000000000000000, -0.000000000000000000, 1.000000000000000000 ) ) ;
#8443=EDGE_LOOP ( 'NONE', ( #4464, #7833, #13814, #8344 ) ) ;
#8462=CARTESIAN_POINT ( 'NONE',  ( -32.07879498588596334, 95.77069236132481933, -15.33800373393474281 ) ) ;
#8465=ADVANCED_FACE ( 'NONE', ( #7653 ), #12442, .F. ) ;
#8473=CARTESIAN_POINT ( 'NONE',  ( -18.52941176470586981, 60.21346111671361001, 26.00000000000000000 ) ) ;
#8474=EDGE_CURVE ( 'NONE', #4578, #2618, #9241, .T. ) ;
#8491=ORIENTED_EDGE ( 'NONE', *, *, #2677, .F. ) ;
#8502=CIRCLE ( 'NONE', #22, 22.00000000000001421 ) ;
#8506=CARTESIAN_POINT ( 'NONE',  ( -11.99241863490640903, 106.3259041464359882, -17.21938144708833462 ) ) ;
#8514=EDGE_CURVE ( 'NONE', #11572, #14934, #6942, .T. ) ;
#8515=VECTOR ( 'NONE', #10198, 1000.000000000000114 ) ;
#8519=ORIENTED_EDGE ( 'NONE', *, *, #532, .F. ) ;
#8525=DIRECTION ( 'NONE',  ( -0.000000000000000000, -0.000000000000000000, 1.000000000000000000 ) ) ;
#8531=EDGE_CURVE ( 'NONE', #10105, #1597, #12360, .T. ) ;
#8538=CARTESIAN_POINT ( 'NONE',  ( 9.442781676091986043, 62.28890912541182701, -19.61600713740890356 ) ) ;
#8544=CARTESIAN_POINT ( 'NONE',  ( 7.500000000000000888, 106.7368258849775202, -20.00000000000000000 ) ) ;
#8545=VECTOR ( 'NONE', #12776, 1000.000000000000000 ) ;
#8577=AXIS2_PLACEMENT_3D ( 'NONE', #14831, #4434, #13689 ) ;
#8582=CARTESIAN_POINT ( 'NONE',  ( 30.68753049492184815, 96.22530292649337014, -14.05553407057507087 ) ) ;
#8584=AXIS2_PLACEMENT_3D ( 'NONE', #10574, #9201, #1172 ) ;
#8591=CARTESIAN_POINT ( 'NONE',  ( 25.00000000000000000, 81.24038404635960831, -23.50000000000000000 ) ) ;
#8594=DIRECTION ( 'NONE',  ( 0.000000000000000000, 0.000000000000000000, -1.000000000000000000 ) ) ;
#8598=ORIENTED_EDGE ( 'NONE', *, *, #11310, .F. ) ;
#8601=DIRECTION ( 'NONE',  ( -0.000000000000000000, -0.000000000000000000, 1.000000000000000000 ) ) ;
#8606=DIRECTION ( 'NONE',  ( 0.000000000000000000, 0.000000000000000000, 1.000000000000000000 ) ) ;
#8617=CARTESIAN_POINT ( 'NONE',  ( -29.86558579037015448, 96.48341332593351183, -12.29240575635728838 ) ) ;
#8619=ORIENTED_EDGE ( 'NONE', *, *, #844, .F. ) ;
#8622=CARTESIAN_POINT ( 'NONE',  ( 0.000000000000000000, 0.000000000000000000, -16.00000000000000000 ) ) ;
#8630=FACE_OUTER_BOUND ( 'NONE', #9179, .T. ) ;
#8632=ORIENTED_EDGE ( 'NONE', *, *, #11770, .T. ) ;
#8634=CARTESIAN_POINT ( 'NONE',  ( 7.500000000000007105, 85.00000000000000000, 46.00000000000000000 ) ) ;
#8641=DIRECTION ( 'NONE',  ( 1.000000000000000000, 0.000000000000000000, 0.000000000000000000 ) ) ;
#8643=CARTESIAN_POINT ( 'NONE',  ( 35.50612649840986990, 100.5723974928649511, -15.96895346309147534 ) ) ;
#8644=CARTESIAN_POINT ( 'NONE',  ( -31.47058823529412663, 102.2673069760056421, -31.00000000000000000 ) ) ;
#8646=DIRECTION ( 'NONE',  ( -1.000000000000000000, 0.000000000000000000, 0.000000000000000000 ) ) ;
#8652=EDGE_CURVE ( 'NONE', #5062, #8404, #11461, .T. ) ;
#8658=CARTESIAN_POINT ( 'NONE',  ( 31.32379180359345838, 96.02017129613331292, -14.76790389961145245 ) ) ;
#8662=LINE ( 'NONE', #2680, #11885 ) ;
#8663=VERTEX_POINT ( 'NONE', #4690 ) ;
#8665=CARTESIAN_POINT ( 'NONE',  ( 11.99241863490641080, 106.3259041464360024, 17.21938144708833462 ) ) ;
#8667=DIRECTION ( 'NONE',  ( -0.000000000000000000, -0.000000000000000000, -1.000000000000000000 ) ) ;
#8683=DIRECTION ( 'NONE',  ( -0.000000000000000000, 0.000000000000000000, 1.000000000000000000 ) ) ;
#8697=CARTESIAN_POINT ( 'NONE',  ( -18.52941176470586981, 60.21346111671361001, -31.00000000000000000 ) ) ;
#8700=AXIS2_PLACEMENT_3D ( 'NONE', #9271, #4511, #1307 ) ;
#8707=( GEOMETRIC_REPRESENTATION_CONTEXT ( 3 ) GLOBAL_UNCERTAINTY_ASSIGNED_CONTEXT ( ( #3987 ) ) GLOBAL_UNIT_ASSIGNED_CONTEXT ( ( #13732, #11455, #7869 ) ) REPRESENTATION_CONTEXT ( 'NONE', 'WORKASPACE' ) );
#8715=DIRECTION ( 'NONE',  ( -1.000000000000000000, 0.000000000000000000, 0.000000000000000000 ) ) ;
#8728=CARTESIAN_POINT ( 'NONE',  ( 34.13789339514568155, 95.05636893381512209, -16.00000000000000355 ) ) ;
#8733=VERTEX_POINT ( 'NONE', #1849 ) ;
#8738=CARTESIAN_POINT ( 'NONE',  ( 11.47554877443044674, 106.3830115231064042, 18.04988257186027312 ) ) ;
#8740=EDGE_CURVE ( 'NONE', #10570, #14085, #4413, .T. ) ;
#8745=CIRCLE ( 'NONE', #5598, 7.500000000000001776 ) ;
#8746=ORIENTED_EDGE ( 'NONE', *, *, #9855, .T. ) ;
#8750=CARTESIAN_POINT ( 'NONE',  ( 12.39897948556635754, 73.96800191783272282, -16.00000000000000000 ) ) ;
#8763=LINE ( 'NONE', #11204, #10233 ) ;
#8766=CARTESIAN_POINT ( 'NONE',  ( -25.00000000000000000, 81.24038404635962252, -26.00000000000000000 ) ) ;
#8768=DIRECTION ( 'NONE',  ( 0.000000000000000000, 0.000000000000000000, -1.000000000000000000 ) ) ;
#8778=EDGE_LOOP ( 'NONE', ( #205, #1276, #2728, #8938 ) ) ;
#8781=VECTOR ( 'NONE', #7002, 1000.000000000000114 ) ;
#8794=CARTESIAN_POINT ( 'NONE',  ( -32.35652065542060285, 95.67730775537752663, 15.49454652436122615 ) ) ;
#8805=ORIENTED_EDGE ( 'NONE', *, *, #13331, .T. ) ;
#8809=AXIS2_PLACEMENT_3D ( 'NONE', #9508, #8525, #412 ) ;
#8819=AXIS2_PLACEMENT_3D ( 'NONE', #2062, #3060, #14677 ) ;
#8823=DIRECTION ( 'NONE',  ( 0.000000000000000000, 0.000000000000000000, -1.000000000000000000 ) ) ;
#8846=CARTESIAN_POINT ( 'NONE',  ( 27.94117647058824616, 90.79807628710781842, 13.50000000000000533 ) ) ;
#8847=DIRECTION ( 'NONE',  ( -0.000000000000000000, -0.000000000000000000, 1.000000000000000000 ) ) ;
#8850=EDGE_CURVE ( 'NONE', #13430, #12536, #6048, .T. ) ;
#8862=AXIS2_PLACEMENT_3D ( 'NONE', #1720, #6325, #10982 ) ;
#8866=CARTESIAN_POINT ( 'NONE',  ( -34.09759333678486115, 101.2734996710205451, 15.50321023462188030 ) ) ;
#8888=EDGE_CURVE ( 'NONE', #508, #5898, #10705, .T. ) ;
#8894=CARTESIAN_POINT ( 'NONE',  ( 5.204748896376250896E-15, 85.00000000000000000, 46.00000000000000000 ) ) ;
#8901=CARTESIAN_POINT ( 'NONE',  ( 12.28339058173379783, 73.98737765342407613, -16.56626766863480782 ) ) ;
#8902=CARTESIAN_POINT ( 'NONE',  ( 12.39897948556635754, 94.18739463280904545, -16.00000000000000000 ) ) ;
#8912=CARTESIAN_POINT ( 'NONE',  ( 10.00086283267470932, 106.5319533799504654, -19.34189422912923462 ) ) ;
#8923=DIRECTION ( 'NONE',  ( -0.000000000000000000, -0.000000000000000000, 1.000000000000000000 ) ) ;
#8930=DIRECTION ( 'NONE',  ( 0.000000000000000000, 0.000000000000000000, -1.000000000000000000 ) ) ;
#8937=PRODUCT_DEFINITION ( 'UNKNOWN', '', #2184, #14586 ) ;
#8938=ORIENTED_EDGE ( 'NONE', *, *, #5337, .F. ) ;
#8945=B_SPLINE_CURVE_WITH_KNOTS ( 'NONE', 3,
 ( #3628, #854, #10603, #2056, #137, #201, #9027, #9112, #3196, #3275 ),
 .UNSPECIFIED., .F., .F.,
 ( 4, 2, 2, 2, 4 ),
 ( 0.000000000000000000, 0.001715760189696190381, 0.003431520379392380762, 0.005147280569088571144, 0.006863040758784761525 ),
 .UNSPECIFIED. ) ;
#8955=ORIENTED_EDGE ( 'NONE', *, *, #699, .F. ) ;
#8958=CARTESIAN_POINT ( 'NONE',  ( 0.000000000000000000, 0.000000000000000000, 16.00000000000000000 ) ) ;
#8964=MANIFOLD_SOLID_BREP ( 'Cavity1', #4074 ) ;
#8968=CARTESIAN_POINT ( 'NONE',  ( 7.500000000000000888, 59.24038404635959409, -15.00000000000000355 ) ) ;
#8971=EDGE_CURVE ( 'NONE', #13514, #2375, #12843, .T. ) ;
#8972=ORIENTED_EDGE ( 'NONE', *, *, #10202, .T. ) ;
#8981=EDGE_CURVE ( 'NONE', #6713, #1920, #2464, .T. ) ;
#8983=VERTEX_POINT ( 'NONE', #2436 ) ;
#8987=CARTESIAN_POINT ( 'NONE',  ( 11.99124924651180102, 106.3260354126052363, -17.22144562113022204 ) ) ;
#8989=SHAPE_DEFINITION_REPRESENTATION ( #13369, #10623 ) ;
#8990=ORIENTED_EDGE ( 'NONE', *, *, #13914, .F. ) ;
#8994=ADVANCED_FACE ( 'NONE', ( #88, #10632 ), #3519, .T. ) ;
#8997=CARTESIAN_POINT ( 'NONE',  ( 33.83495342806090633, 101.3902949203995689, 15.35262818605211699 ) ) ;
#8999=ORIENTED_EDGE ( 'NONE', *, *, #6018, .T. ) ;
#9001=ORIENTED_EDGE ( 'NONE', *, *, #9855, .F. ) ;
#9007=DIRECTION ( 'NONE',  ( 1.000000000000000000, 6.308085367188385311E-16, 0.000000000000000000 ) ) ;
#9027=CARTESIAN_POINT ( 'NONE',  ( 11.47656068366043414, 61.94660012053729048, 18.08543280684388321 ) ) ;
#9045=AXIS2_PLACEMENT_3D ( 'NONE', #9213, #6856, #13711 ) ;
#9048=CARTESIAN_POINT ( 'NONE',  ( 11.46115996437298712, 94.30629603967057051, -18.06445797889986338 ) ) ;
#9062=CARTESIAN_POINT ( 'NONE',  ( 47.00000000000001421, 81.24038404635960831, 31.00000000000000000 ) ) ;
#9064=VERTEX_POINT ( 'NONE', #10568 ) ;
#9069=CARTESIAN_POINT ( 'NONE',  ( 12.39897948556635576, 94.18739463280904545, 16.00000000000000000 ) ) ;
#9070=AXIS2_PLACEMENT_3D ( 'NONE', #10300, #3323, #2104 ) ;
#9074=EDGE_LOOP ( 'NONE', ( #5597, #13866 ) ) ;
#9076=CIRCLE ( 'NONE', #13953, 17.00000000000001066 ) ;
#9079=AXIS2_PLACEMENT_3D ( 'NONE', #12191, #1711, #4072 ) ;
#9084=SHAPE_REPRESENTATION_RELATIONSHIP ( 'NONE' , 'NONE' ,  #10623, #2938 ) ;
#9097=ORIENTED_EDGE ( 'NONE', *, *, #13546, .F. ) ;
#9098=DIRECTION ( 'NONE',  ( 0.000000000000000000, 0.000000000000000000, 1.000000000000000000 ) ) ;
#9107=CARTESIAN_POINT ( 'NONE',  ( -25.00000000000000000, 81.24038404635962252, 16.00000000000000000 ) ) ;
#9112=CARTESIAN_POINT ( 'NONE',  ( 12.07479981346994258, 61.83277384271320187, 17.09860361742227397 ) ) ;
#9116=B_SPLINE_CURVE_WITH_KNOTS ( 'NONE', 3,
 ( #8399, #13108, #2854, #428, #8617, #6026, #578, #7239, #5134, #5210, #14247, #14314, #13036, #8462, #7404, #14475, #9525, #11983, #4077, #13187 ),
 .UNSPECIFIED., .F., .F.,
 ( 4, 2, 2, 2, 2, 2, 2, 2, 2, 4 ),
 ( 0.000000000000000000, 0.0009765910691878001981, 0.001464886603781702466, 0.001953182138375604733, 0.002929773207563409268, 0.003906364276751213803, 0.004882955345939018338, 0.005859546415126822873, 0.006836137484314629142, 0.007812728553502436279 ),
 .UNSPECIFIED. ) ;
#9117=CARTESIAN_POINT ( 'NONE',  ( 34.44830544488820578, 94.94374256356070418, 16.00000000000000000 ) ) ;
#9121=DIRECTION ( 'NONE',  ( 1.000000000000000000, 0.000000000000000000, 0.000000000000000000 ) ) ;
#9122=CIRCLE ( 'NONE', #638, 4.999999999999995559 ) ;
#9128=( LENGTH_UNIT ( ) NAMED_UNIT ( * ) SI_UNIT ( .MILLI., .METRE. ) );
#9149=CARTESIAN_POINT ( 'NONE',  ( 32.45630819848047111, 101.9391205390361250, 14.06872601623944696 ) ) ;
#9165=AXIS2_PLACEMENT_3D ( 'NONE', #135, #200, #10830 ) ;
#9166=ADVANCED_FACE ( 'NONE', ( #11015 ), #12086, .F. ) ;
#9173=EDGE_CURVE ( 'NONE', #8983, #5358, #13150, .T. ) ;
#9179=EDGE_LOOP ( 'NONE', ( #4736, #12753, #7721, #7231 ) ) ;
#9181=EDGE_CURVE ( 'NONE', #10382, #11572, #10937, .T. ) ;
#9187=CARTESIAN_POINT ( 'NONE',  ( -10.19763225997207101, 62.16969414240132608, 19.21937000502254023 ) ) ;
#9192=FACE_OUTER_BOUND ( 'NONE', #12656, .T. ) ;
#9201=DIRECTION ( 'NONE',  ( -0.000000000000000000, -0.000000000000000000, 1.000000000000000000 ) ) ;
#9208=ORIENTED_EDGE ( 'NONE', *, *, #10712, .F. ) ;
#9209=AXIS2_PLACEMENT_3D ( 'NONE', #11412, #10266, #14907 ) ;
#9213=CARTESIAN_POINT ( 'NONE',  ( -25.00000000000000000, 81.24038404635962252, -31.00000000000000000 ) ) ;
#9216=AXIS2_PLACEMENT_3D ( 'NONE', #2687, #7302, #11959 ) ;
#9217=CARTESIAN_POINT ( 'NONE',  ( -12.39897948556635754, 61.76783392443436327, -16.00000000000000000 ) ) ;
#9233=VECTOR ( 'NONE', #2946, 1000.000000000000000 ) ;
#9237=ORIENTED_EDGE ( 'NONE', *, *, #8474, .F. ) ;
#9241=CIRCLE ( 'NONE', #3919, 95.00000000000001421 ) ;
#9245=ORIENTED_EDGE ( 'NONE', *, *, #1702, .T. ) ;
#9246=DIRECTION ( 'NONE',  ( 1.000000000000000000, 0.000000000000000000, 0.000000000000000000 ) ) ;
#9263=AXIS2_PLACEMENT_3D ( 'NONE', #8591, #5038, #2757 ) ;
#9265=CARTESIAN_POINT ( 'NONE',  ( -11.08335940112994855, 62.01770010158976731, 18.49860775790518730 ) ) ;
#9269=CARTESIAN_POINT ( 'NONE',  ( -10.80089892394231832, 106.4537193389066374, 18.76964747820619905 ) ) ;
#9270=CARTESIAN_POINT ( 'NONE',  ( -27.94117647058823550, 90.79807628710781842, -23.50000000000000000 ) ) ;
#9271=CARTESIAN_POINT ( 'NONE',  ( 0.000000000000000000, 0.000000000000000000, -26.00000000000000000 ) ) ;
#9278=CARTESIAN_POINT ( 'NONE',  ( 7.500000000000000888, 94.70348462437907244, -20.00000000000000000 ) ) ;
#9281=AXIS2_PLACEMENT_3D ( 'NONE', #4440, #10350, #13852 ) ;
#9285=CYLINDRICAL_SURFACE ( 'NONE', #2551, 22.00000000000000355 ) ;
#9287=DIRECTION ( 'NONE',  ( 1.000000000000000000, 0.000000000000000000, 0.000000000000000000 ) ) ;
#9291=ORIENTED_EDGE ( 'NONE', *, *, #14471, .F. ) ;
#9302=SURFACE_SIDE_STYLE ('',( #3472 ) ) ;
#9305=CIRCLE ( 'NONE', #99, 5.000000000000001776 ) ;
#9312=DIRECTION ( 'NONE',  ( 0.000000000000000000, 0.000000000000000000, -1.000000000000000000 ) ) ;
#9320=AXIS2_PLACEMENT_3D ( 'NONE', #13032, #8315, #10593 ) ;
#9321=EDGE_LOOP ( 'NONE', ( #11267, #9896, #7065, #12508, #14955, #13240, #2323, #4465 ) ) ;
#9325=CARTESIAN_POINT ( 'NONE',  ( 25.00000000000000000, 81.24038404635960831, 16.00000000000000000 ) ) ;
#9327=CARTESIAN_POINT ( 'NONE',  ( -11.62988759722695953, 74.09296836101485439, -17.83282915334323349 ) ) ;
#9331=CIRCLE ( 'NONE', #8121, 17.00000000000000711 ) ;
#9347=DIRECTION ( 'NONE',  ( 0.000000000000000000, 0.000000000000000000, 1.000000000000000000 ) ) ;
#9350=CARTESIAN_POINT ( 'NONE',  ( -12.46748823216054625, 106.2711901036691273, -15.65608700630148675 ) ) ;
#9351=CARTESIAN_POINT ( 'NONE',  ( 8.636355552181207429, 94.60704768011227372, -19.87755835258713688 ) ) ;
#9358=LINE ( 'NONE', #2235, #7295 ) ;
#9363=DIRECTION ( 'NONE',  ( -0.000000000000000000, -0.000000000000000000, -1.000000000000000000 ) ) ;
#9375=LINE ( 'NONE', #47, #6553 ) ;
#9381=ORIENTED_EDGE ( 'NONE', *, *, #4912, .F. ) ;
#9383=DIRECTION ( 'NONE',  ( 0.000000000000000000, 0.000000000000000000, 1.000000000000000000 ) ) ;
#9389=EDGE_CURVE ( 'NONE', #1392, #11614, #8745, .T. ) ;
#9390=CARTESIAN_POINT ( 'NONE',  ( -19.99999999999998934, 64.99230723708770086, -26.00000000000000000 ) ) ;
#9393=DIRECTION ( 'NONE',  ( 1.000000000000000000, 0.000000000000000000, 0.000000000000000000 ) ) ;
#9395=DIRECTION ( 'NONE',  ( 0.2941176470588241498, -0.9557692240748186796, 0.000000000000000000 ) ) ;
#9404=ORIENTED_EDGE ( 'NONE', *, *, #1928, .F. ) ;
#9408=CARTESIAN_POINT ( 'NONE',  ( -10.00086283267471465, 106.5319533799504939, 19.34189422912923817 ) ) ;
#9411=CARTESIAN_POINT ( 'NONE',  ( 25.00000000000000000, 81.24038404635960831, 13.50000000000000533 ) ) ;
#9421=ORIENTED_EDGE ( 'NONE', *, *, #9181, .T. ) ;
#9438=TOROIDAL_SURFACE ( 'NONE', #3383, 17.00000000000001066, 5.000000000000000000 ) ;
#9442=CARTESIAN_POINT ( 'NONE',  ( 12.50000000000000000, 106.2673515243510991, 15.00000000000000000 ) ) ;
#9448=CIRCLE ( 'NONE', #6525, 95.00000000000001421 ) ;
#9468=CARTESIAN_POINT ( 'NONE',  ( 0.000000000000000000, 0.000000000000000000, 20.00000000000000000 ) ) ;
#9470=CARTESIAN_POINT ( 'NONE',  ( -12.26010588040893978, 73.99122283359872654, -16.55683232866783783 ) ) ;
#9471=VECTOR ( 'NONE', #2192, 1000.000000000000000 ) ;
#9473=ORIENTED_EDGE ( 'NONE', *, *, #9389, .T. ) ;
#9477=EDGE_CURVE ( 'NONE', #10382, #6653, #12152, .T. ) ;
#9482=CARTESIAN_POINT ( 'NONE',  ( 31.47058823529413374, 102.2673069760056563, 31.00000000000000000 ) ) ;
#9483=FACE_OUTER_BOUND ( 'NONE', #1290, .T. ) ;
#9485=CARTESIAN_POINT ( 'NONE',  ( 12.50000000000000000, 100.2235002382176248, -15.00000000000000000 ) ) ;
#9489=DIRECTION ( 'NONE',  ( 1.000000000000000000, 0.000000000000000000, -0.000000000000000000 ) ) ;
#9490=AXIS2_PLACEMENT_3D ( 'NONE', #11190, #11266, #8823 ) ;
#9501=ORIENTED_EDGE ( 'NONE', *, *, #7365, .F. ) ;
#9506=CARTESIAN_POINT ( 'NONE',  ( -19.99999999999998934, 64.99230723708770086, -31.00000000000000000 ) ) ;
#9508=CARTESIAN_POINT ( 'NONE',  ( 25.00000000000000000, 81.24038404635960831, -23.50000000000000000 ) ) ;
#9515=B_SPLINE_CURVE_WITH_KNOTS ( 'NONE', 3,
 ( #6191, #7247, #9530, #1722 ),
 .UNSPECIFIED., .F., .F.,
 ( 4, 4 ),
 ( 3.469446951953614189E-18, 0.001005167940839970337 ),
 .UNSPECIFIED. ) ;
#9516=ADVANCED_FACE ( 'NONE', ( #3727 ), #1740, .F. ) ;
#9517=ORIENTED_EDGE ( 'NONE', *, *, #3287, .T. ) ;
#9518=AXIS2_PLACEMENT_3D ( 'NONE', #9827, #8768, #12117 ) ;
#9522=CARTESIAN_POINT ( 'NONE',  ( 8.156204789939931032, 106.6891793314720331, 19.96764982490488904 ) ) ;
#9525=CARTESIAN_POINT ( 'NONE',  ( -33.22084910410213610, 95.38070844757929478, -15.83879782491089117 ) ) ;
#9530=CARTESIAN_POINT ( 'NONE',  ( 12.46631608856921325, 100.2277185551817809, -15.67011936326128918 ) ) ;
#9539=MECHANICAL_DESIGN_GEOMETRIC_PRESENTATION_REPRESENTATION('',(#5347),#8707);
#9547=CARTESIAN_POINT ( 'NONE',  ( 7.500000000000000888, 59.24038404635959409, -15.00000000000000355 ) ) ;
#9555=DIRECTION ( 'NONE',  ( 0.000000000000000000, 0.000000000000000000, 1.000000000000000000 ) ) ;
#9568=ORIENTED_EDGE ( 'NONE', *, *, #3839, .T. ) ;
#9579=DIRECTION ( 'NONE',  ( 0.9557692240748190127, -0.2941176470588235392, 0.000000000000000000 ) ) ;
#9584=CARTESIAN_POINT ( 'NONE',  ( -31.50188236243966244, 102.2577520262375685, -11.65984174646773219 ) ) ;
#9590=CARTESIAN_POINT ( 'NONE',  ( 12.39897948556635754, 100.2360479454198696, -16.00000000000000000 ) ) ;
#9606=DIRECTION ( 'NONE',  ( 0.000000000000000000, 0.000000000000000000, -1.000000000000000000 ) ) ;
#9614=VERTEX_POINT ( 'NONE', #9924 ) ;
#9622=ORIENTED_EDGE ( 'NONE', *, *, #3242, .T. ) ;
#9629=LINE ( 'NONE', #8644, #11032 ) ;
#9646=CARTESIAN_POINT ( 'NONE',  ( -34.65532077583675630, 101.0090414146251447, -15.74457401924681044 ) ) ;
#9647=CYLINDRICAL_SURFACE ( 'NONE', #8809, 10.00000000000000178 ) ;
#9648=CARTESIAN_POINT ( 'NONE',  ( 0.000000000000000000, 0.000000000000000000, 16.00000000000000000 ) ) ;
#9653=DIRECTION ( 'NONE',  ( -0.000000000000000000, -0.000000000000000000, 1.000000000000000000 ) ) ;
#9655=EDGE_CURVE ( 'NONE', #6159, #1593, #3390, .T. ) ;
#9657=CARTESIAN_POINT ( 'NONE',  ( 29.70588235294119173, 96.53269163155674448, -10.99999999999999645 ) ) ;
#9668=AXIS2_PLACEMENT_3D ( 'NONE', #2198, #2281, #5761 ) ;
#9685=ORIENTED_EDGE ( 'NONE', *, *, #8740, .T. ) ;
#9691=ORIENTED_EDGE ( 'NONE', *, *, #12502, .F. ) ;
#9696=ADVANCED_FACE ( 'NONE', ( #5259 ), #1466, .F. ) ;
#9704=CIRCLE ( 'NONE', #3182, 107.0000000000000284 ) ;
#9726=CARTESIAN_POINT ( 'NONE',  ( -25.00000000000000000, 81.24038404635962252, -31.00000000000000000 ) ) ;
#9731=CARTESIAN_POINT ( 'NONE',  ( 12.50000000000000000, 106.2673515243510991, 15.00000000000000000 ) ) ;
#9766=ORIENTED_EDGE ( 'NONE', *, *, #8850, .T. ) ;
#9776=CYLINDRICAL_SURFACE ( 'NONE', #10036, 5.000000000000000000 ) ;
#9787=EDGE_CURVE ( 'NONE', #12536, #7623, #8662, .T. ) ;
#9792=EDGE_LOOP ( 'NONE', ( #13757, #1166, #7704, #827 ) ) ;
#9801=CARTESIAN_POINT ( 'NONE',  ( 12.23689275498546536, 106.2979809871390415, 16.60898801976832573 ) ) ;
#9803=CARTESIAN_POINT ( 'NONE',  ( 5.000000000000007105, 85.00000000000000000, 46.00000000000000000 ) ) ;
#9815=EDGE_CURVE ( 'NONE', #721, #13514, #10897, .T. ) ;
#9816=CARTESIAN_POINT ( 'NONE',  ( -29.70588235294118107, 96.53269163155674448, -79.80561291909842225 ) ) ;
#9823=ORIENTED_EDGE ( 'NONE', *, *, #2165, .T. ) ;
#9825=CARTESIAN_POINT ( 'NONE',  ( -12.07490296461408974, 74.02221379130672574, 17.09816637537096540 ) ) ;
#9826=CARTESIAN_POINT ( 'NONE',  ( 7.500000000000000000, 106.7368258849775202, 20.00000000000000355 ) ) ;
#9827=CARTESIAN_POINT ( 'NONE',  ( 12.50000000000000000, 40.62019202317980415, -31.00000000000000000 ) ) ;
#9828=CARTESIAN_POINT ( 'NONE',  ( -12.50000000000000000, 40.62019202317981126, 23.50000000000000355 ) ) ;
#9829=EDGE_LOOP ( 'NONE', ( #10140, #1651, #5602, #3964, #5689, #2792, #4014, #8805, #5224, #650, #13985 ) ) ;
#9832=AXIS2_PLACEMENT_3D ( 'NONE', #2016, #12426, #4235 ) ;
#9842=DIRECTION ( 'NONE',  ( -1.000000000000000000, 0.000000000000000000, 0.000000000000000000 ) ) ;
#9847=CARTESIAN_POINT ( 'NONE',  ( -31.72333741318944433, 102.1879147510518919, 12.61437971294004790 ) ) ;
#9854=CARTESIAN_POINT ( 'NONE',  ( 18.52941176470587692, 60.21346111671358159, 26.00000000000000000 ) ) ;
#9855=EDGE_CURVE ( 'NONE', #14546, #10333, #4842, .T. ) ;
#9857=DIRECTION ( 'NONE',  ( -0.000000000000000000, -0.000000000000000000, 1.000000000000000000 ) ) ;
#9886=PLANE ( 'NONE',  #7851 ) ;
#9896=ORIENTED_EDGE ( 'NONE', *, *, #11310, .T. ) ;
#9904=DIRECTION ( 'NONE',  ( -0.9557692240748190127, -0.2941176470588235392, -5.100557892117772022E-16 ) ) ;
#9912=ORIENTED_EDGE ( 'NONE', *, *, #8110, .F. ) ;
#9924=CARTESIAN_POINT ( 'NONE',  ( 5.000000000000007105, 85.00000000000000000, 31.00000000000000000 ) ) ;
#9929=CARTESIAN_POINT ( 'NONE',  ( -32.78625152019765920, 95.53054288192238630, 15.68243957109766207 ) ) ;
#9930=CIRCLE ( 'NONE', #3396, 7.500000000000001776 ) ;
#9948=CARTESIAN_POINT ( 'NONE',  ( 32.35652065542060285, 95.67730775537752663, -15.49454652436121727 ) ) ;
#9949=ORIENTED_EDGE ( 'NONE', *, *, #13441, .F. ) ;
#9952=ORIENTED_EDGE ( 'NONE', *, *, #10847, .T. ) ;
#9955=VERTEX_POINT ( 'NONE', #1905 ) ;
#9964=EDGE_CURVE ( 'NONE', #13797, #7984, #4025, .T. ) ;
#9968=CARTESIAN_POINT ( 'NONE',  ( 12.50000000000000000, 40.62019202317980415, 31.00000000000000000 ) ) ;
#9978=ORIENTED_EDGE ( 'NONE', *, *, #8531, .F. ) ;
#9991=EDGE_CURVE ( 'NONE', #1689, #8733, #4870, .T. ) ;
#9997=CARTESIAN_POINT ( 'NONE',  ( -12.50000000000000000, 100.2235002382176248, -15.33678752976415716 ) ) ;
#10002=CARTESIAN_POINT ( 'NONE',  ( 25.00000000000000000, 81.24038404635960831, 26.00000000000000000 ) ) ;
#10003=CARTESIAN_POINT ( 'NONE',  ( -33.82975856321728969, 101.3925934381291256, 15.34957766734057927 ) ) ;
#10007=EDGE_CURVE ( 'NONE', #7249, #8663, #994, .T. ) ;
#10011=CARTESIAN_POINT ( 'NONE',  ( -30.88479107129467849, 96.16227383530475947, 14.30703002621670095 ) ) ;
#10014=AXIS2_PLACEMENT_3D ( 'NONE', #3392, #5592, #10224 ) ;
#10036=AXIS2_PLACEMENT_3D ( 'NONE', #10160, #4414, #845 ) ;
#10046=AXIS2_PLACEMENT_3D ( 'NONE', #646, #7458, #6097 ) ;
#10052=ORIENTED_EDGE ( 'NONE', *, *, #4809, .T. ) ;
#10054=DIRECTION ( 'NONE',  ( -0.2941176470588238168, 0.9557692240748187906, -0.000000000000000000 ) ) ;
#10064=ORIENTED_EDGE ( 'NONE', *, *, #7306, .T. ) ;
#10075=ORIENTED_EDGE ( 'NONE', *, *, #10285, .T. ) ;
#10076=B_SPLINE_CURVE_WITH_KNOTS ( 'NONE', 3,
 ( #1670, #14347, #3954, #8355, #7431, #1447, #10707, #12079, #6276, #12997, #10925, #531, #14272, #2585, #4032, #2657, #310, #8643, #7275, #13284 ),
 .UNSPECIFIED., .F., .F.,
 ( 4, 2, 2, 2, 2, 2, 2, 2, 2, 4 ),
 ( 0.000000000000000000, 0.0009815662899613894401, 0.001472349434942086871, 0.001963132579922784084, 0.002944698869884174175, 0.003926265159845563832, 0.004907831449806954356, 0.005889397739768344013, 0.006870964029729732803, 0.007852530319691122460 ),
 .UNSPECIFIED. ) ;
#10077=CARTESIAN_POINT ( 'NONE',  ( -12.39897948556635754, 100.2360479454198696, 16.00000000000000000 ) ) ;
#10080=CARTESIAN_POINT ( 'NONE',  ( -12.50000000000000000, 100.2235002382176248, 15.00000000000000000 ) ) ;
#10105=VERTEX_POINT ( 'NONE', #4869 ) ;
#10106=CARTESIAN_POINT ( 'NONE',  ( 34.44830544488820578, 94.94374256356071839, -16.00000000000000000 ) ) ;
#10107=CARTESIAN_POINT ( 'NONE',  ( 0.000000000000000000, 0.000000000000000000, -26.00000000000000000 ) ) ;
#10109=CARTESIAN_POINT ( 'NONE',  ( -11.62509980388830577, 61.91833518448029849, 17.84018927347701933 ) ) ;
#10111=CARTESIAN_POINT ( 'NONE',  ( -8.075974454121990220, 94.65787058575050139, -19.99999999999999289 ) ) ;
#10115=CARTESIAN_POINT ( 'NONE',  ( -15.11621636258860946, 32.12188890498260463, 11.00000000000000000 ) ) ;
#10119=CARTESIAN_POINT ( 'NONE',  ( 10.88232432232082125, 94.37491168429329491, -18.69329470938989957 ) ) ;
#10125=DIRECTION ( 'NONE',  ( 0.000000000000000000, 0.000000000000000000, -1.000000000000000000 ) ) ;
#10126=CARTESIAN_POINT ( 'NONE',  ( 7.500000000000000000, 74.62405778299650194, 20.00000000000000000 ) ) ;
#10128=VECTOR ( 'NONE', #4550, 1000.000000000000000 ) ;
#10137=CARTESIAN_POINT ( 'NONE',  ( 36.08010649850015739, 100.2464683348682541, 16.00000000000000000 ) ) ;
#10140=ORIENTED_EDGE ( 'NONE', *, *, #10285, .F. ) ;
#10142=CARTESIAN_POINT ( 'NONE',  ( -12.46631608856921325, 100.2277185551817809, 15.67011936326128563 ) ) ;
#10151=EDGE_CURVE ( 'NONE', #6653, #5203, #453, .T. ) ;
#10159=ORIENTED_EDGE ( 'NONE', *, *, #5931, .F. ) ;
#10160=CARTESIAN_POINT ( 'NONE',  ( -36.24943435566822103, 100.7967187407115262, -10.99999999999999645 ) ) ;
#10163=ORIENTED_EDGE ( 'NONE', *, *, #5316, .F. ) ;
#10173=ORIENTED_EDGE ( 'NONE', *, *, #3242, .F. ) ;
#10174=CARTESIAN_POINT ( 'NONE',  ( 33.22084910410213610, 95.38070844757928057, 15.83879782491088761 ) ) ;
#10178=CARTESIAN_POINT ( 'NONE',  ( -9.719110480984905820, 94.50309565249440880, -19.51732164073033715 ) ) ;
#10186=PLANE ( 'NONE',  #8577 ) ;
#10197=ORIENTED_EDGE ( 'NONE', *, *, #5708, .F. ) ;
#10198=DIRECTION ( 'NONE',  ( 0.2941176470588243164, 0.9557692240748185686, -0.000000000000000000 ) ) ;
#10202=EDGE_CURVE ( 'NONE', #1809, #5665, #10076, .T. ) ;
#10203=AXIS2_PLACEMENT_3D ( 'NONE', #1594, #379, #10918 ) ;
#10204=ORIENTED_EDGE ( 'NONE', *, *, #3771, .T. ) ;
#10215=DIRECTION ( 'NONE',  ( 0.000000000000000000, 0.000000000000000000, 1.000000000000000000 ) ) ;
#10222=CARTESIAN_POINT ( 'NONE',  ( 12.34196858416779996, 73.97755844198597686, 16.27929523640516862 ) ) ;
#10224=DIRECTION ( 'NONE',  ( 1.000000000000000000, 0.000000000000000000, 0.000000000000000000 ) ) ;
#10227=VECTOR ( 'NONE', #8208, 1000.000000000000000 ) ;
#10233=VECTOR ( 'NONE', #10054, 1000.000000000000114 ) ;
#10237=EDGE_CURVE ( 'NONE', #4479, #13246, #7726, .T. ) ;
#10252=CIRCLE ( 'NONE', #3221, 10.00000000000000355 ) ;
#10257=ADVANCED_FACE ( 'NONE', ( #14583 ), #4186, .F. ) ;
#10263=VECTOR ( 'NONE', #9606, 1000.000000000000000 ) ;
#10264=CARTESIAN_POINT ( 'NONE',  ( -10.21436410913239357, 94.45034564433045432, -19.23824501837257017 ) ) ;
#10265=LINE ( 'NONE', #6978, #261 ) ;
#10266=DIRECTION ( 'NONE',  ( -0.9557692240748187906, -0.2941176470588238168, 0.000000000000000000 ) ) ;
#10268=CYLINDRICAL_SURFACE ( 'NONE', #2517, 5.000000000000000888 ) ;
#10281=FACE_OUTER_BOUND ( 'NONE', #11906, .T. ) ;
#10284=CARTESIAN_POINT ( 'NONE',  ( 7.500000000000000888, 106.7368258849775202, -20.00000000000000000 ) ) ;
#10285=EDGE_CURVE ( 'NONE', #5509, #8172, #6064, .T. ) ;
#10292=CARTESIAN_POINT ( 'NONE',  ( 35.08068705722487124, 100.7955773171491813, 15.87635720896652458 ) ) ;
#10293=LINE ( 'NONE', #2385, #8781 ) ;
#10298=ORIENTED_EDGE ( 'NONE', *, *, #3477, .F. ) ;
#10299=AXIS2_PLACEMENT_3D ( 'NONE', #6702, #3152, #885 ) ;
#10300=CARTESIAN_POINT ( 'NONE',  ( -12.50000000000000000, 59.24038404635959409, 20.00000000000000000 ) ) ;
#10310=LINE ( 'NONE', #2180, #4730 ) ;
#10315=VERTEX_POINT ( 'NONE', #4334 ) ;
#10319=VECTOR ( 'NONE', #13553, 1000.000000000000000 ) ;
#10320=DIRECTION ( 'NONE',  ( 0.2941176470588243164, 0.9557692240748185686, 0.000000000000000000 ) ) ;
#10322=CIRCLE ( 'NONE', #1833, 75.00000000000001421 ) ;
#10333=VERTEX_POINT ( 'NONE', #5536 ) ;
#10339=CARTESIAN_POINT ( 'NONE',  ( -12.50000000000000000, 106.2673515243510991, 15.00000000000000000 ) ) ;
#10340=CYLINDRICAL_SURFACE ( 'NONE', #5403, 10.00000000000000178 ) ;
#10350=DIRECTION ( 'NONE',  ( -0.9557692240748187906, 0.2941176470588240388, 0.000000000000000000 ) ) ;
#10361=ORIENTED_EDGE ( 'NONE', *, *, #8217, .F. ) ;
#10367=ADVANCED_FACE ( 'NONE', ( #10465 ), #11471, .T. ) ;
#10372=ADVANCED_FACE ( 'NONE', ( #4705 ), #3336, .T. ) ;
#10375=DIRECTION ( 'NONE',  ( -0.000000000000000000, 1.000000000000000000, -0.000000000000000000 ) ) ;
#10376=SURFACE_STYLE_USAGE ( .BOTH. , #9302 ) ;
#10381=EDGE_LOOP ( 'NONE', ( #868, #3319, #13158, #14558, #8424 ) ) ;
#10382=VERTEX_POINT ( 'NONE', #13974 ) ;
#10384=CARTESIAN_POINT ( 'NONE',  ( 20.00000000000000000, 64.99230723708768664, 31.00000000000000000 ) ) ;
#10385=ORIENTED_EDGE ( 'NONE', *, *, #686, .T. ) ;
#10401=ORIENTED_EDGE ( 'NONE', *, *, #11282, .T. ) ;
#10405=B_SPLINE_CURVE_WITH_KNOTS ( 'NONE', 3,
 ( #11045, #4133, #4062, #12105, #11116, #6536, #13390, #14459, #8901, #8750 ),
 .UNSPECIFIED., .F., .F.,
 ( 4, 2, 2, 2, 4 ),
 ( 0.000000000000000000, 0.001711864931188371644, 0.003423729862376743288, 0.005135594793565114932, 0.006847459724753486576 ),
 .UNSPECIFIED. ) ;
#10408=DIRECTION ( 'NONE',  ( -0.000000000000000000, -0.000000000000000000, 1.000000000000000000 ) ) ;
#10411=CIRCLE ( 'NONE', #4124, 22.00000000000001421 ) ;
#10419=ORIENTED_EDGE ( 'NONE', *, *, #3525, .T. ) ;
#10430=DIRECTION ( 'NONE',  ( 0.000000000000000000, 0.000000000000000000, -1.000000000000000000 ) ) ;
#10441=ORIENTED_EDGE ( 'NONE', *, *, #3331, .T. ) ;
#10454=EDGE_CURVE ( 'NONE', #10950, #4578, #8036, .T. ) ;
#10460=VECTOR ( 'NONE', #3366, 1000.000000000000114 ) ;
#10465=FACE_OUTER_BOUND ( 'NONE', #6924, .T. ) ;
#10474=ORIENTED_EDGE ( 'NONE', *, *, #13785, .F. ) ;
#10490=EDGE_CURVE ( 'NONE', #2772, #14249, #5601, .T. ) ;
#10493=CARTESIAN_POINT ( 'NONE',  ( -10.55213320575001923, 106.4787665061024313, -18.97395805252363843 ) ) ;
#10506=CARTESIAN_POINT ( 'NONE',  ( 12.50000000000000000, 40.62019202317980415, 16.00000000000000000 ) ) ;
#10510=CARTESIAN_POINT ( 'NONE',  ( 25.00000000000000000, 81.24038404635960831, 26.00000000000000000 ) ) ;
#10511=LINE ( 'NONE', #2461, #2539 ) ;
#10527=CARTESIAN_POINT ( 'NONE',  ( -10.44268084954785714, 94.42456965614839248, 19.05230465901501091 ) ) ;
#10531=PLANE ( 'NONE',  #9165 ) ;
#10534=CIRCLE ( 'NONE', #5460, 95.00000000000001421 ) ;
#10540=DIRECTION ( 'NONE',  ( 0.9557692240748186796, 0.2941176470588241498, 1.531423350357148967E-16 ) ) ;
#10541=CARTESIAN_POINT ( 'NONE',  ( -11.10403672352021331, 74.17481381252333961, 18.51301757891051025 ) ) ;
#10544=CARTESIAN_POINT ( 'NONE',  ( -9.706343076449424956, 74.36968214894433515, -19.49591231693629112 ) ) ;
#10546=EDGE_LOOP ( 'NONE', ( #8148, #1659, #9237, #1219, #10052, #9291, #13475, #383 ) ) ;
#10553=ADVANCED_FACE ( 'NONE', ( #7336 ), #1508, .F. ) ;
#10558=ORIENTED_EDGE ( 'NONE', *, *, #8474, .T. ) ;
#10568=CARTESIAN_POINT ( 'NONE',  ( -18.52941176470586981, 60.21346111671361001, 16.00000000000000000 ) ) ;
#10570=VERTEX_POINT ( 'NONE', #2720 ) ;
#10572=CARTESIAN_POINT ( 'NONE',  ( 8.072481656125567895, 94.65682832148054615, -19.97535367358596403 ) ) ;
#10574=CARTESIAN_POINT ( 'NONE',  ( 0.000000000000000000, 0.000000000000000000, -31.00000000000000000 ) ) ;
#10586=AXIS2_PLACEMENT_3D ( 'NONE', #9968, #1780, #6692 ) ;
#10593=DIRECTION ( 'NONE',  ( 1.000000000000000000, 0.000000000000000000, 0.000000000000000000 ) ) ;
#10603=CARTESIAN_POINT ( 'NONE',  ( 8.635061085254619684, 62.40781208424768778, 19.90323072647615632 ) ) ;
#10609=CARTESIAN_POINT ( 'NONE',  ( -12.39897948556635754, 73.96800191783272282, 16.00000000000000000 ) ) ;
#10610=ADVANCED_FACE ( 'NONE', ( #8630 ), #12961, .T. ) ;
#10616=CYLINDRICAL_SURFACE ( 'NONE', #842, 5.000000000000001776 ) ;
#10623=SHAPE_REPRESENTATION ( 'brake caliper housing', ( #5108 ), #14072 ) ;
#10626=CARTESIAN_POINT ( 'NONE',  ( -10.43254889841015220, 62.13061131512488089, 19.05984907584256760 ) ) ;
#10632=FACE_BOUND ( 'NONE', #3638, .T. ) ;
#10637=EDGE_CURVE ( 'NONE', #6344, #4010, #14171, .T. ) ;
#10642=ORIENTED_EDGE ( 'NONE', *, *, #8850, .F. ) ;
#10647=FACE_OUTER_BOUND ( 'NONE', #8443, .T. ) ;
#10648=EDGE_CURVE ( 'NONE', #1542, #10333, #3038, .T. ) ;
#10649=ORIENTED_EDGE ( 'NONE', *, *, #12893, .F. ) ;
#10653=DIRECTION ( 'NONE',  ( 1.000000000000000000, 0.000000000000000000, 0.000000000000000000 ) ) ;
#10658=ORIENTED_EDGE ( 'NONE', *, *, #9173, .T. ) ;
#10661=CARTESIAN_POINT ( 'NONE',  ( 8.801203450618841018, 106.6379082728991534, 19.83890680725671274 ) ) ;
#10663=VECTOR ( 'NONE', #9857, 1000.000000000000000 ) ;
#10674=B_SPLINE_CURVE_WITH_KNOTS ( 'NONE', 3,
 ( #4850, #6754, #9470, #12981, #8264, #9327, #14116, #7191, #6689, #3572, #11844, #10544, #5492, #8189, #12552, #2414, #3723, #12479 ),
 .UNSPECIFIED., .F., .F.,
 ( 4, 2, 2, 2, 2, 2, 2, 2, 4 ),
 ( 0.001002962753164631828, 0.001858089309406474668, 0.002713215865648317508, 0.003568342421890159915, 0.004423468978132002322, 0.005278595534373845162, 0.006133722090615688002, 0.006988848646857530843, 0.007843975203099373683 ),
 .UNSPECIFIED. ) ;
#10677=CARTESIAN_POINT ( 'NONE',  ( 20.00000000000000000, 64.99230723708768664, -31.00000000000000000 ) ) ;
#10695=CIRCLE ( 'NONE', #6806, 5.000000000000001776 ) ;
#10699=EDGE_CURVE ( 'NONE', #1593, #508, #6392, .T. ) ;
#10705=CIRCLE ( 'NONE', #9490, 5.000000000000000888 ) ;
#10707=CARTESIAN_POINT ( 'NONE',  ( 31.77701906416544020, 102.1706497334997721, -12.77113345645743792 ) ) ;
#10712=EDGE_CURVE ( 'NONE', #1597, #11013, #11723, .T. ) ;
#10757=CARTESIAN_POINT ( 'NONE',  ( 19.99999999999999645, 64.99230723708767243, 26.00000000000000000 ) ) ;
#10758=ORIENTED_EDGE ( 'NONE', *, *, #11602, .T. ) ;
#10762=EDGE_CURVE ( 'NONE', #2772, #5947, #5226, .T. ) ;
#10768=DIRECTION ( 'NONE',  ( 1.000000000000000000, 0.000000000000000000, 0.000000000000000000 ) ) ;
#10772=ORIENTED_EDGE ( 'NONE', *, *, #12158, .F. ) ;
#10783=DIRECTION ( 'NONE',  ( 1.000000000000000000, 0.000000000000000000, 0.000000000000000000 ) ) ;
#10793=ADVANCED_FACE ( 'NONE', ( #5667 ), #11372, .T. ) ;
#10797=CARTESIAN_POINT ( 'NONE',  ( 12.50000000000000000, 59.24038404635959409, 20.00000000000000000 ) ) ;
#10800=ORIENTED_EDGE ( 'NONE', *, *, #3078, .F. ) ;
#10813=CARTESIAN_POINT ( 'NONE',  ( -11.46115996437298357, 94.30629603967057051, 18.06445797889986338 ) ) ;
#10830=DIRECTION ( 'NONE',  ( -1.000000000000000000, 0.000000000000000000, -0.000000000000000000 ) ) ;
#10835=ORIENTED_EDGE ( 'NONE', *, *, #13081, .F. ) ;
#10842=ORIENTED_EDGE ( 'NONE', *, *, #13396, .F. ) ;
#10847=EDGE_CURVE ( 'NONE', #5358, #13983, #467, .T. ) ;
#10848=ADVANCED_FACE ( 'NONE', ( #7865 ), #4483, .T. ) ;
#10870=ORIENTED_EDGE ( 'NONE', *, *, #5708, .T. ) ;
#10873=CARTESIAN_POINT ( 'NONE',  ( -7.500000000000000888, 106.7368258849775202, 20.00000000000000355 ) ) ;
#10876=ORIENTED_EDGE ( 'NONE', *, *, #10648, .F. ) ;
#10885=EDGE_CURVE ( 'NONE', #1920, #6713, #3516, .T. ) ;
#10897=B_SPLINE_CURVE_WITH_KNOTS ( 'NONE', 3,
 ( #6227, #405, #6162, #470 ),
 .UNSPECIFIED., .F., .F.,
 ( 4, 4 ),
 ( 0.000000000000000000, 0.001005167940839974024 ),
 .UNSPECIFIED. ) ;
#10905=CARTESIAN_POINT ( 'NONE',  ( 0.000000000000000000, 0.000000000000000000, -16.00000000000000000 ) ) ;
#10909=DIRECTION ( 'NONE',  ( 0.000000000000000000, 0.000000000000000000, 1.000000000000000000 ) ) ;
#10918=DIRECTION ( 'NONE',  ( 1.000000000000000000, -4.440892098500626162E-15, 0.000000000000000000 ) ) ;
#10925=CARTESIAN_POINT ( 'NONE',  ( 32.65070903206050446, 101.8685403450051155, -14.31792419690431650 ) ) ;
#10929=EDGE_CURVE ( 'NONE', #2375, #7147, #94, .T. ) ;
#10932=DIRECTION ( 'NONE',  ( 0.000000000000000000, -1.000000000000000000, 0.000000000000000000 ) ) ;
#10937=LINE ( 'NONE', #14437, #11671 ) ;
#10943=VERTEX_POINT ( 'NONE', #7168 ) ;
#10944=DIRECTION ( 'NONE',  ( -0.000000000000000000, -0.000000000000000000, -1.000000000000000000 ) ) ;
#10945=EDGE_LOOP ( 'NONE', ( #3785, #1025, #2978, #6269 ) ) ;
#10950=VERTEX_POINT ( 'NONE', #10952 ) ;
#10951=EDGE_CURVE ( 'NONE', #3168, #2447, #5184, .T. ) ;
#10952=CARTESIAN_POINT ( 'NONE',  ( -7.500000000000000888, 106.7368258849775202, -20.00000000000000000 ) ) ;
#10963=CYLINDRICAL_SURFACE ( 'NONE', #10046, 22.00000000000001421 ) ;
#10964=LINE ( 'NONE', #9816, #12200 ) ;
#10971=CARTESIAN_POINT ( 'NONE',  ( -7.500000000000000888, 59.24038404635959409, -15.00000000000000000 ) ) ;
#10973=CARTESIAN_POINT ( 'NONE',  ( 0.000000000000000000, 0.000000000000000000, -20.00000000000000000 ) ) ;
#10976=CARTESIAN_POINT ( 'NONE',  ( 31.47058823529413374, 102.2673069760056563, -10.99999999999999645 ) ) ;
#10980=CIRCLE ( 'NONE', #3469, 10.00000000000000178 ) ;
#10982=DIRECTION ( 'NONE',  ( 0.000000000000000000, 0.000000000000000000, 1.000000000000000000 ) ) ;
#10994=EDGE_CURVE ( 'NONE', #6159, #7414, #12017, .T. ) ;
#10998=CARTESIAN_POINT ( 'NONE',  ( -33.32140965599871407, 101.6077678005751324, 14.98557208302583632 ) ) ;
#11005=CARTESIAN_POINT ( 'NONE',  ( -32.93386454278234510, 95.47976343162785895, 15.73819668677757910 ) ) ;
#11013=VERTEX_POINT ( 'NONE', #3066 ) ;
#11014=AXIS2_PLACEMENT_3D ( 'NONE', #11490, #5623, #1087 ) ;
#11015=FACE_OUTER_BOUND ( 'NONE', #6498, .T. ) ;
#11017=FACE_OUTER_BOUND ( 'NONE', #11459, .T. ) ;
#11024=CARTESIAN_POINT ( 'NONE',  ( 32.93386454278233799, 95.47976343162785895, -15.73819668677757555 ) ) ;
#11032=VECTOR ( 'NONE', #6140, 1000.000000000000000 ) ;
#11043=EDGE_LOOP ( 'NONE', ( #3334, #10842, #14163, #12952 ) ) ;
#11045=CARTESIAN_POINT ( 'NONE',  ( 7.500000000000000888, 74.62405778299650194, -20.00000000000000000 ) ) ;
#11057=CARTESIAN_POINT ( 'NONE',  ( 12.28299834225913045, 61.79111542428975667, -16.56818924177462904 ) ) ;
#11069=EDGE_CURVE ( 'NONE', #4578, #10105, #4084, .T. ) ;
#11083=CARTESIAN_POINT ( 'NONE',  ( -30.68753049492183749, 96.22530292649338435, 14.05553407057507620 ) ) ;
#11106=CARTESIAN_POINT ( 'NONE',  ( 12.18091848848563608, 106.3044177073317087, 16.76518324937863014 ) ) ;
#11116=CARTESIAN_POINT ( 'NONE',  ( 10.21287289150292743, 74.30275811153845211, -19.23918552186209041 ) ) ;
#11118=B_SPLINE_CURVE_WITH_KNOTS ( 'NONE', 3,
 ( #762, #4184, #684, #12223, #450, #11005, #9929, #8794, #1820, #613, #2810, #10011, #11083, #6273, #13432, #3040, #7660, #5079, #12303, #5391 ),
 .UNSPECIFIED., .F., .F.,
 ( 4, 2, 2, 2, 2, 2, 2, 2, 2, 4 ),
 ( 0.000000000000000000, 0.0009765940263104732309, 0.001464891039465707027, 0.001953188052620940824, 0.002929782078931390202, 0.003906376105241839147, 0.004882970131552281587, 0.005859564157862724894, 0.006836158184173168201, 0.007812752210483610640 ),
 .UNSPECIFIED. ) ;
#11122=CARTESIAN_POINT ( 'NONE',  ( 25.00000000000000000, 81.24038404635960831, -16.00000000000000000 ) ) ;
#11134=CARTESIAN_POINT ( 'NONE',  ( -47.00000000000000000, 81.24038404635962252, -26.00000000000000000 ) ) ;
#11140=ORIENTED_EDGE ( 'NONE', *, *, #14471, .T. ) ;
#11159=AXIS2_PLACEMENT_3D ( 'NONE', #6279, #10932, #7280 ) ;
#11164=CARTESIAN_POINT ( 'NONE',  ( 0.000000000000000000, 0.000000000000000000, 20.00000000000000355 ) ) ;
#11169=ADVANCED_FACE ( 'NONE', ( #9483 ), #1225, .T. ) ;
#11190=CARTESIAN_POINT ( 'NONE',  ( -42.00000000000000000, 81.24038404635962252, -26.00000000000000000 ) ) ;
#11195=FACE_OUTER_BOUND ( 'NONE', #3624, .T. ) ;
#11202=STYLED_ITEM ( 'NONE', ( #13533 ), #8964 ) ;
#11204=CARTESIAN_POINT ( 'NONE',  ( -31.47058823529412663, 102.2673069760056563, 10.99999999999999645 ) ) ;
#11205=CARTESIAN_POINT ( 'NONE',  ( 10.54368182729040093, 106.4795995572428353, -18.98024639174784056 ) ) ;
#11209=ORIENTED_EDGE ( 'NONE', *, *, #9815, .F. ) ;
#11212=DIRECTION ( 'NONE',  ( 0.2941176470588237613, -0.9557692240748189016, 0.000000000000000000 ) ) ;
#11214=LINE ( 'NONE', #818, #1791 ) ;
#11217=ADVANCED_FACE ( 'NONE', ( #7129 ), #14056, .T. ) ;
#11219=ORIENTED_EDGE ( 'NONE', *, *, #14530, .T. ) ;
#11220=ORIENTED_EDGE ( 'NONE', *, *, #3543, .T. ) ;
#11234=VERTEX_POINT ( 'NONE', #3813 ) ;
#11237=ORIENTED_EDGE ( 'NONE', *, *, #7115, .T. ) ;
#11246=EDGE_LOOP ( 'NONE', ( #10197, #3368, #1421, #6723, #12104, #12297, #4105, #8746, #10419 ) ) ;
#11252=DIRECTION ( 'NONE',  ( 1.000000000000000000, 0.000000000000000000, 0.000000000000000000 ) ) ;
#11263=AXIS2_PLACEMENT_3D ( 'NONE', #13981, #1292, #11416 ) ;
#11266=DIRECTION ( 'NONE',  ( -0.000000000000000000, -1.000000000000000000, -0.000000000000000000 ) ) ;
#11267=ORIENTED_EDGE ( 'NONE', *, *, #1294, .F. ) ;
#11270=AXIS2_PLACEMENT_3D ( 'NONE', #6620, #1654, #6258 ) ;
#11274=AXIS2_PLACEMENT_3D ( 'NONE', #5148, #1586, #1429 ) ;
#11279=FACE_OUTER_BOUND ( 'NONE', #1618, .T. ) ;
#11282=EDGE_CURVE ( 'NONE', #1593, #14956, #9629, .T. ) ;
#11289=CIRCLE ( 'NONE', #10299, 75.00000000000001421 ) ;
#11290=AXIS2_PLACEMENT_3D ( 'NONE', #3986, #8601, #2843 ) ;
#11292=ORIENTED_EDGE ( 'NONE', *, *, #8981, .F. ) ;
#11295=DIRECTION ( 'NONE',  ( -0.000000000000000000, -0.000000000000000000, 1.000000000000000000 ) ) ;
#11308=FACE_OUTER_BOUND ( 'NONE', #9829, .T. ) ;
#11309=CARTESIAN_POINT ( 'NONE',  ( -32.10455955028197650, 102.0624585623582021, 13.51511155787192031 ) ) ;
#11310=EDGE_CURVE ( 'NONE', #4446, #4839, #7133, .T. ) ;
#11342=DIRECTION ( 'NONE',  ( 0.000000000000000000, 1.000000000000000000, 0.000000000000000000 ) ) ;
#11355=CARTESIAN_POINT ( 'NONE',  ( 12.50000000000000000, 106.2673515243510991, -15.00000000000000355 ) ) ;
#11363=CARTESIAN_POINT ( 'NONE',  ( 9.719110480984905820, 94.50309565249440880, 19.51732164073033715 ) ) ;
#11372=PLANE ( 'NONE',  #9070 ) ;
#11373=ADVANCED_FACE ( 'NONE', ( #5024 ), #9776, .F. ) ;
#11374=DIRECTION ( 'NONE',  ( 1.000000000000000000, 0.000000000000000000, 0.000000000000000000 ) ) ;
#11387=ORIENTED_EDGE ( 'NONE', *, *, #2903, .T. ) ;
#11397=CARTESIAN_POINT ( 'NONE',  ( 0.000000000000000000, 0.000000000000000000, 25.99999999999999645 ) ) ;
#11406=CARTESIAN_POINT ( 'NONE',  ( -11.45661564179884628, 61.94983405580221358, 18.07016506142803891 ) ) ;
#11412=CARTESIAN_POINT ( 'NONE',  ( -31.47058823529412663, 102.2673069760056563, -79.80561291909842225 ) ) ;
#11416=DIRECTION ( 'NONE',  ( -0.9557692240748183465, 0.2941176470588252045, 0.000000000000000000 ) ) ;
#11424=AXIS2_PLACEMENT_3D ( 'NONE', #7356, #5165, #3656 ) ;
#11430=LINE ( 'NONE', #882, #10460 ) ;
#11435=AXIS2_PLACEMENT_3D ( 'NONE', #9390, #10540, #3796 ) ;
#11436=CARTESIAN_POINT ( 'NONE',  ( 9.104688129943030006, 106.6120509519917192, -19.73833377876427519 ) ) ;
#11439=VECTOR ( 'NONE', #4102, 1000.000000000000000 ) ;
#11451=CARTESIAN_POINT ( 'NONE',  ( 8.635752201752492141, 74.50170565226535757, 19.87768552833457392 ) ) ;
#11452=PRODUCT ( 'brake caliper housing', 'brake caliper housing', '', ( #7056 ) ) ;
#11455=( NAMED_UNIT ( * ) PLANE_ANGLE_UNIT ( ) SI_UNIT ( $, .RADIAN. ) );
#11459=EDGE_LOOP ( 'NONE', ( #3714, #730, #465, #5183 ) ) ;
#11461=LINE ( 'NONE', #3327, #14585 ) ;
#11471=PLANE ( 'NONE',  #2197 ) ;
#11483=DIRECTION ( 'NONE',  ( -0.000000000000000000, -0.000000000000000000, 1.000000000000000000 ) ) ;
#11490=CARTESIAN_POINT ( 'NONE',  ( 0.000000000000000000, 0.000000000000000000, -16.00000000000000000 ) ) ;
#11494=CARTESIAN_POINT ( 'NONE',  ( -7.500000000000000888, 106.7368258849775202, 20.00000000000000355 ) ) ;
#11507=B_SPLINE_CURVE_WITH_KNOTS ( 'NONE', 3,
 ( #10106, #8728, #5321, #6595, #5482, #11024, #629, #9948, #12167, #857, #8658, #3970, #8582, #7510, #2891, #13375, #777, #6516, #7595, #2829 ),
 .UNSPECIFIED., .F., .F.,
 ( 4, 2, 2, 2, 2, 2, 2, 2, 2, 4 ),
 ( 0.000000000000000000, 0.0009765940263104426564, 0.001464891039465661274, 0.001953188052620879675, 0.002929782078931332957, 0.003906376105241786238, 0.004882970131552239086, 0.005859564157862691934, 0.006836158184173144782, 0.007812752210483598497 ),
 .UNSPECIFIED. ) ;
#11517=DIRECTION ( 'NONE',  ( -1.000000000000000000, 0.000000000000000000, 0.000000000000000000 ) ) ;
#11526=CIRCLE ( 'NONE', #4965, 95.00000000000001421 ) ;
#11535=CIRCLE ( 'NONE', #12733, 17.00000000000000711 ) ;
#11538=FACE_OUTER_BOUND ( 'NONE', #1371, .T. ) ;
#11539=FACE_OUTER_BOUND ( 'NONE', #11589, .T. ) ;
#11545=DIRECTION ( 'NONE',  ( 1.000000000000000000, 0.000000000000000000, 0.000000000000000000 ) ) ;
#11556=AXIS2_PLACEMENT_3D ( 'NONE', #12450, #9098, #9246 ) ;
#11566=B_SPLINE_CURVE_WITH_KNOTS ( 'NONE', 3,
 ( #8902, #1852, #13536, #3143, #7760, #2000, #9048, #5496, #10119, #14762, #4359, #7836, #13696, #2520, #9351, #10572, #5715, #9278 ),
 .UNSPECIFIED., .F., .F.,
 ( 4, 2, 2, 2, 2, 2, 2, 2, 4 ),
 ( 0.001002887730653551817, 0.001856445934617264627, 0.002710004138580977221, 0.003563562342544689815, 0.004417120546508402842, 0.005270678750472115003, 0.006124236954435828030, 0.006977795158399540190, 0.007831353362363253218 ),
 .UNSPECIFIED. ) ;
#11572=VERTEX_POINT ( 'NONE', #4559 ) ;
#11574=ORIENTED_EDGE ( 'NONE', *, *, #530, .T. ) ;
#11575=DIRECTION ( 'NONE',  ( 0.000000000000000000, 0.000000000000000000, -1.000000000000000000 ) ) ;
#11576=DIRECTION ( 'NONE',  ( -0.000000000000000000, -0.000000000000000000, 1.000000000000000000 ) ) ;
#11578=LINE ( 'NONE', #4510, #7754 ) ;
#11589=EDGE_LOOP ( 'NONE', ( #7945, #11574, #10401, #1118, #804, #6487, #7157, #13556 ) ) ;
#11596=DIRECTION ( 'NONE',  ( 0.000000000000000000, 0.000000000000000000, -1.000000000000000000 ) ) ;
#11602=EDGE_CURVE ( 'NONE', #14105, #8983, #4267, .T. ) ;
#11603=DIRECTION ( 'NONE',  ( 0.000000000000000000, 0.000000000000000000, 1.000000000000000000 ) ) ;
#11612=DIRECTION ( 'NONE',  ( 0.2941176470588243164, 0.9557692240748186796, -0.000000000000000000 ) ) ;
#11614=VERTEX_POINT ( 'NONE', #13977 ) ;
#11631=CARTESIAN_POINT ( 'NONE',  ( 31.32121808728250656, 96.02101045561127535, 14.76552927760548073 ) ) ;
#11636=DIRECTION ( 'NONE',  ( -0.000000000000000000, -0.000000000000000000, 1.000000000000000000 ) ) ;
#11640=AXIS2_PLACEMENT_3D ( 'NONE', #9107, #4711, #12762 ) ;
#11645=CARTESIAN_POINT ( 'NONE',  ( -25.00000000000000000, 81.24038404635962252, 26.00000000000000000 ) ) ;
#11646=DIRECTION ( 'NONE',  ( -1.000000000000000000, 0.000000000000000000, 0.000000000000000000 ) ) ;
#11650=ORIENTED_EDGE ( 'NONE', *, *, #12475, .T. ) ;
#11663=VECTOR ( 'NONE', #5081, 1000.000000000000000 ) ;
#11667=CIRCLE ( 'NONE', #2916, 10.00000000000000178 ) ;
#11669=EDGE_LOOP ( 'NONE', ( #7781, #2282, #10800, #14835, #14861, #8619 ) ) ;
#11671=VECTOR ( 'NONE', #12020, 1000.000000000000000 ) ;
#11678=VECTOR ( 'NONE', #6178, 1000.000000000000000 ) ;
#11686=DIRECTION ( 'NONE',  ( -1.000000000000000000, 0.000000000000000000, 0.000000000000000000 ) ) ;
#11700=DIRECTION ( 'NONE',  ( 0.000000000000000000, 0.000000000000000000, 1.000000000000000000 ) ) ;
#11707=ORIENTED_EDGE ( 'NONE', *, *, #515, .T. ) ;
#11713=CARTESIAN_POINT ( 'NONE',  ( -8.632958377326437116, 106.6512898904676092, 19.87266383408973525 ) ) ;
#11714=FACE_OUTER_BOUND ( 'NONE', #14069, .T. ) ;
#11723=B_SPLINE_CURVE_WITH_KNOTS ( 'NONE', 3,
 ( #1876, #672, #9997, #6645 ),
 .UNSPECIFIED., .F., .F.,
 ( 4, 4 ),
 ( 0.000000000000000000, 0.001005167940839974024 ),
 .UNSPECIFIED. ) ;
#11735=ORIENTED_EDGE ( 'NONE', *, *, #12903, .T. ) ;
#11744=ORIENTED_EDGE ( 'NONE', *, *, #7590, .F. ) ;
#11755=CARTESIAN_POINT ( 'NONE',  ( -12.34206246762915882, 94.19488728021195811, 16.27883530325393835 ) ) ;
#11758=CARTESIAN_POINT ( 'NONE',  ( 0.000000000000000000, 0.000000000000000000, -16.00000000000000000 ) ) ;
#11770=EDGE_CURVE ( 'NONE', #13905, #5260, #9305, .T. ) ;
#11775=CARTESIAN_POINT ( 'NONE',  ( -12.39897948556635754, 73.96800191783273704, -16.00000000000000000 ) ) ;
#11782=EDGE_LOOP ( 'NONE', ( #3258, #3616, #9421, #138, #10361 ) ) ;
#11790=DIRECTION ( 'NONE',  ( 1.000000000000000000, -7.105427357601001859E-15, 0.000000000000000000 ) ) ;
#11792=DIRECTION ( 'NONE',  ( -1.000000000000000000, 0.000000000000000000, 0.000000000000000000 ) ) ;
#11834=VERTEX_POINT ( 'NONE', #673 ) ;
#11843=DIRECTION ( 'NONE',  ( -0.000000000000000000, -0.000000000000000000, 1.000000000000000000 ) ) ;
#11844=CARTESIAN_POINT ( 'NONE',  ( -10.20278626552728873, 74.30320229487229255, -19.21617406370430103 ) ) ;
#11846=CARTESIAN_POINT ( 'NONE',  ( 25.00000000000000000, 81.24038404635960831, -26.00000000000000000 ) ) ;
#11848=ADVANCED_FACE ( 'NONE', ( #1808 ), #3173, .T. ) ;
#11853=CARTESIAN_POINT ( 'NONE',  ( -30.00000000000000711, 97.48846085563154418, 31.00000000000000000 ) ) ;
#11855=CARTESIAN_POINT ( 'NONE',  ( 0.000000000000000000, 0.000000000000000000, 26.00000000000000000 ) ) ;
#11863=CARTESIAN_POINT ( 'NONE',  ( -12.50000000000000000, 106.2673515243511133, -15.33083626825422918 ) ) ;
#11865=LINE ( 'NONE', #11949, #1057 ) ;
#11870=ORIENTED_EDGE ( 'NONE', *, *, #10007, .T. ) ;
#11878=CARTESIAN_POINT ( 'NONE',  ( -35.79345569434273244, 100.4135791079098112, -16.00000000000000355 ) ) ;
#11885=VECTOR ( 'NONE', #14227, 1000.000000000000000 ) ;
#11902=B_SPLINE_CURVE_WITH_KNOTS ( 'NONE', 3,
 ( #10137, #3316, #736, #10292, #6559, #14858, #4533, #3164, #8997, #3091, #7785, #2098, #9149, #4236, #6636, #7636, #12505, #12284, #6711, #13720 ),
 .UNSPECIFIED., .F., .F.,
 ( 4, 2, 2, 2, 2, 2, 2, 2, 2, 4 ),
 ( 0.000000000000000000, 0.0009816351435713618467, 0.001472452715357043746, 0.001963270287142725428, 0.002944905430714073180, 0.003926540574285420498, 0.004908175717856767817, 0.005889810861428116003, 0.006871446004999463321, 0.007853081148570811507 ),
 .UNSPECIFIED. ) ;
#11906=EDGE_LOOP ( 'NONE', ( #4689, #8182, #1645, #3969, #12193, #4048 ) ) ;
#11920=EDGE_CURVE ( 'NONE', #12353, #5584, #12928, .T. ) ;
#11930=ORIENTED_EDGE ( 'NONE', *, *, #3605, .F. ) ;
#11934=FACE_OUTER_BOUND ( 'NONE', #12907, .T. ) ;
#11945=APPLICATION_CONTEXT ( 'automotive_design' ) ;
#11946=DIRECTION ( 'NONE',  ( 0.000000000000000000, 0.000000000000000000, 1.000000000000000000 ) ) ;
#11948=CARTESIAN_POINT ( 'NONE',  ( -12.50000000000000000, 106.2673515243510991, -15.00000000000000000 ) ) ;
#11949=CARTESIAN_POINT ( 'NONE',  ( 29.70588235294119173, 96.53269163155674448, -10.99999999999999645 ) ) ;
#11955=VERTEX_POINT ( 'NONE', #970 ) ;
#11959=DIRECTION ( 'NONE',  ( 1.000000000000000000, 0.000000000000000000, 0.000000000000000000 ) ) ;
#11969=EDGE_CURVE ( 'NONE', #7984, #143, #12660, .T. ) ;
#11983=CARTESIAN_POINT ( 'NONE',  ( -33.83031011230892915, 95.16624652083667968, -15.96768307234233397 ) ) ;
#11990=LINE ( 'NONE', #12059, #10263 ) ;
#12009=EDGE_LOOP ( 'NONE', ( #1361, #6919, #12391, #7486 ) ) ;
#12017=CIRCLE ( 'NONE', #369, 102.0000000000000142 ) ;
#12020=DIRECTION ( 'NONE',  ( 0.000000000000000000, 0.000000000000000000, -1.000000000000000000 ) ) ;
#12022=ADVANCED_FACE ( 'NONE', ( #6871 ), #12880, .F. ) ;
#12024=ADVANCED_FACE ( 'NONE', ( #11539, #48 ), #8090, .T. ) ;
#12059=CARTESIAN_POINT ( 'NONE',  ( 12.50000000000000000, 106.2673515243510991, -31.00000000000000000 ) ) ;
#12079=CARTESIAN_POINT ( 'NONE',  ( 31.95756590787640050, 102.1116157579503181, -13.22695225398608088 ) ) ;
#12086=CYLINDRICAL_SURFACE ( 'NONE', #6784, 101.0000000000000284 ) ;
#12094=EDGE_LOOP ( 'NONE', ( #3160, #1637, #14559, #3234 ) ) ;
#12097=DIRECTION ( 'NONE',  ( -0.000000000000000000, -1.000000000000000000, -0.000000000000000000 ) ) ;
#12101=CARTESIAN_POINT ( 'NONE',  ( -35.08068705722485703, 100.7955773171491813, -15.87635720896652103 ) ) ;
#12104=ORIENTED_EDGE ( 'NONE', *, *, #14880, .T. ) ;
#12105=CARTESIAN_POINT ( 'NONE',  ( 9.718176292668216476, 74.36971601906103047, -19.51774219187060311 ) ) ;
#12111=CIRCLE ( 'NONE', #1681, 101.0000000000000284 ) ;
#12116=CARTESIAN_POINT ( 'NONE',  ( 9.703618315745391243, 62.24871376222710495, -19.49715125027359974 ) ) ;
#12117=DIRECTION ( 'NONE',  ( -1.000000000000000000, 0.000000000000000000, -0.000000000000000000 ) ) ;
#12122=FACE_OUTER_BOUND ( 'NONE', #822, .T. ) ;
#12127=ORIENTED_EDGE ( 'NONE', *, *, #7723, .F. ) ;
#12130=CYLINDRICAL_SURFACE ( 'NONE', #13627, 10.00000000000000178 ) ;
#12135=AXIS2_PLACEMENT_3D ( 'NONE', #2756, #9579, #2607 ) ;
#12152=CIRCLE ( 'NONE', #10203, 107.0000000000000284 ) ;
#12158=EDGE_CURVE ( 'NONE', #11013, #1542, #6248, .T. ) ;
#12163=CARTESIAN_POINT ( 'NONE',  ( -7.500000000000000888, 74.62405778299650194, 20.00000000000000000 ) ) ;
#12167=CARTESIAN_POINT ( 'NONE',  ( 32.08430773043614437, 95.76884182151505343, -15.34120815717649222 ) ) ;
#12176=CARTESIAN_POINT ( 'NONE',  ( -36.08010649850015028, 100.2464683348682541, -16.00000000000000000 ) ) ;
#12191=CARTESIAN_POINT ( 'NONE',  ( 25.00000000000000000, 81.24038404635960831, 16.00000000000000000 ) ) ;
#12192=CARTESIAN_POINT ( 'NONE',  ( -12.28339058173379783, 73.98737765342407613, 16.56626766863481137 ) ) ;
#12193=ORIENTED_EDGE ( 'NONE', *, *, #8234, .T. ) ;
#12200=VECTOR ( 'NONE', #14461, 1000.000000000000000 ) ;
#12205=DIRECTION ( 'NONE',  ( -1.000000000000000000, 0.000000000000000000, 0.000000000000000000 ) ) ;
#12212=CARTESIAN_POINT ( 'NONE',  ( -25.00000000000000000, 81.24038404635962252, -26.00000000000000000 ) ) ;
#12223=CARTESIAN_POINT ( 'NONE',  ( -33.38013186279886924, 95.32466787866006541, 15.87266497586409919 ) ) ;
#12225=AXIS2_PLACEMENT_3D ( 'NONE', #3639, #1015, #9395 ) ;
#12234=CIRCLE ( 'NONE', #7614, 101.0000000000000284 ) ;
#12244=ADVANCED_FACE ( 'NONE', ( #3002 ), #576, .T. ) ;
#12249=CIRCLE ( 'NONE', #13190, 107.0000000000000284 ) ;
#12284=CARTESIAN_POINT ( 'NONE',  ( 31.50188236243967665, 102.2577520262375828, 11.65984174646773930 ) ) ;
#12285=DIRECTION ( 'NONE',  ( 0.000000000000000000, 0.000000000000000000, -1.000000000000000000 ) ) ;
#12287=ORIENTED_EDGE ( 'NONE', *, *, #8531, .T. ) ;
#12294=CARTESIAN_POINT ( 'NONE',  ( -12.39897948556635754, 100.2360479454198696, -16.00000000000000000 ) ) ;
#12295=CARTESIAN_POINT ( 'NONE',  ( 12.50000000000000000, 40.62019202317980415, 16.00000000000000000 ) ) ;
#12297=ORIENTED_EDGE ( 'NONE', *, *, #8217, .T. ) ;
#12303=CARTESIAN_POINT ( 'NONE',  ( -29.70588235294120238, 96.53269163155678712, 11.33021639467930797 ) ) ;
#12305=CARTESIAN_POINT ( 'NONE',  ( 0.000000000000000000, 0.000000000000000000, 16.00000000000000000 ) ) ;
#12317=DIRECTION ( 'NONE',  ( -1.000000000000000000, 0.000000000000000000, 0.000000000000000000 ) ) ;
#12335=DIRECTION ( 'NONE',  ( 0.000000000000000000, 0.000000000000000000, -1.000000000000000000 ) ) ;
#12343=DIRECTION ( 'NONE',  ( -0.000000000000000000, -0.000000000000000000, 1.000000000000000000 ) ) ;
#12345=ORIENTED_EDGE ( 'NONE', *, *, #2481, .F. ) ;
#12353=VERTEX_POINT ( 'NONE', #659 ) ;
#12360=LINE ( 'NONE', #1958, #1968 ) ;
#12361=ORIENTED_EDGE ( 'NONE', *, *, #3839, .F. ) ;
#12363=ORIENTED_EDGE ( 'NONE', *, *, #13081, .T. ) ;
#12367=DIRECTION ( 'NONE',  ( 0.000000000000000000, -1.000000000000000000, 0.000000000000000000 ) ) ;
#12373=CARTESIAN_POINT ( 'NONE',  ( 22.05882352941176094, 71.68269180561141241, -23.50000000000000000 ) ) ;
#12384=ORIENTED_EDGE ( 'NONE', *, *, #10885, .F. ) ;
#12391=ORIENTED_EDGE ( 'NONE', *, *, #6354, .F. ) ;
#12400=SURFACE_SIDE_STYLE ('',( #12482 ) ) ;
#12403=FACE_OUTER_BOUND ( 'NONE', #9074, .T. ) ;
#12426=DIRECTION ( 'NONE',  ( -0.000000000000000000, 1.000000000000000000, 0.000000000000000000 ) ) ;
#12438=FILL_AREA_STYLE_COLOUR ( '', #988 ) ;
#12439=CARTESIAN_POINT ( 'NONE',  ( -31.47058823529412663, 102.2673069760056421, -26.00000000000000000 ) ) ;
#12442=PLANE ( 'NONE',  #4895 ) ;
#12450=CARTESIAN_POINT ( 'NONE',  ( 25.00000000000000000, 81.24038404635960831, 26.00000000000000000 ) ) ;
#12452=DIRECTION ( 'NONE',  ( -0.000000000000000000, -0.000000000000000000, -1.000000000000000000 ) ) ;
#12469=ORIENTED_EDGE ( 'NONE', *, *, #6501, .F. ) ;
#12471=CARTESIAN_POINT ( 'NONE',  ( -12.39897948556635754, 94.18739463280904545, -16.00000000000000000 ) ) ;
#12475=EDGE_CURVE ( 'NONE', #8389, #9955, #5574, .T. ) ;
#12479=CARTESIAN_POINT ( 'NONE',  ( -7.500000000000000000, 74.62405778299650194, -20.00000000000000000 ) ) ;
#12482=SURFACE_STYLE_FILL_AREA ( #7832 ) ;
#12484=CARTESIAN_POINT ( 'NONE',  ( 7.500000000000000888, 94.70348462437907244, -20.00000000000000000 ) ) ;
#12494=ORIENTED_EDGE ( 'NONE', *, *, #4809, .F. ) ;
#12498=CARTESIAN_POINT ( 'NONE',  ( 12.33783400350010950, 106.2863213744706172, -16.30550365830425719 ) ) ;
#12502=EDGE_CURVE ( 'NONE', #14249, #5898, #5892, .T. ) ;
#12505=CARTESIAN_POINT ( 'NONE',  ( 31.62605012285506945, 102.2189371620064833, 12.30800327571618880 ) ) ;
#12508=ORIENTED_EDGE ( 'NONE', *, *, #14880, .F. ) ;
#12513=DIRECTION ( 'NONE',  ( -0.000000000000000000, -0.000000000000000000, 1.000000000000000000 ) ) ;
#12518=ORIENTED_EDGE ( 'NONE', *, *, #4427, .T. ) ;
#12532=ADVANCED_FACE ( 'NONE', ( #10647 ), #9647, .F. ) ;
#12536=VERTEX_POINT ( 'NONE', #14297 ) ;
#12550=DIRECTION ( 'NONE',  ( -0.000000000000000000, -0.000000000000000000, 1.000000000000000000 ) ) ;
#12552=CARTESIAN_POINT ( 'NONE',  ( -8.635752201752492141, 74.50170565226535757, -19.87768552833457392 ) ) ;
#12556=DIRECTION ( 'NONE',  ( -1.000000000000000000, 0.000000000000000000, 0.000000000000000000 ) ) ;
#12564=ORIENTED_EDGE ( 'NONE', *, *, #9787, .T. ) ;
#12571=ORIENTED_EDGE ( 'NONE', *, *, #2124, .T. ) ;
#12580=CARTESIAN_POINT ( 'NONE',  ( 11.08463629228402603, 74.17659209477393745, 18.49742775384897087 ) ) ;
#12588=DIRECTION ( 'NONE',  ( -0.000000000000000000, -0.000000000000000000, 1.000000000000000000 ) ) ;
#12593=CARTESIAN_POINT ( 'NONE',  ( -7.500000000000000888, 61.74746958378133144, -20.00000000000000000 ) ) ;
#12609=CARTESIAN_POINT ( 'NONE',  ( 7.500000000000007105, 85.00000000000000000, 46.00000000000000000 ) ) ;
#12617=AXIS2_PLACEMENT_3D ( 'NONE', #12836, #1302, #5 ) ;
#12625=ORIENTED_EDGE ( 'NONE', *, *, #7259, .T. ) ;
#12635=ORIENTED_EDGE ( 'NONE', *, *, #902, .F. ) ;
#12656=EDGE_LOOP ( 'NONE', ( #7718, #10758, #5702, #4166 ) ) ;
#12658=CARTESIAN_POINT ( 'NONE',  ( 8.072319373765147077, 74.56485781596312279, 19.97535925451852989 ) ) ;
#12659=CYLINDRICAL_SURFACE ( 'NONE', #3901, 95.00000000000001421 ) ;
#12660=LINE ( 'NONE', #13731, #8313 ) ;
#12670=CYLINDRICAL_SURFACE ( 'NONE', #681, 101.0000000000000284 ) ;
#12672=EDGE_LOOP ( 'NONE', ( #3295, #755, #8491, #12127, #9208, #9978 ) ) ;
#12692=CARTESIAN_POINT ( 'NONE',  ( 33.83031011230895047, 95.16624652083665126, 15.96768307234234108 ) ) ;
#12694=CIRCLE ( 'NONE', #2751, 10.00000000000000355 ) ;
#12696=CARTESIAN_POINT ( 'NONE',  ( -8.154413083459852274, 106.6893057894985617, 19.96764870088428623 ) ) ;
#12697=DIRECTION ( 'NONE',  ( -0.000000000000000000, -0.000000000000000000, 1.000000000000000000 ) ) ;
#12703=DIRECTION ( 'NONE',  ( 1.000000000000000000, 0.000000000000000000, 0.000000000000000000 ) ) ;
#12723=CIRCLE ( 'NONE', #11014, 95.00000000000001421 ) ;
#12733=AXIS2_PLACEMENT_3D ( 'NONE', #5443, #10215, #14635 ) ;
#12736=CARTESIAN_POINT ( 'NONE',  ( 11.62988759722695953, 74.09296836101485439, 17.83282915334323349 ) ) ;
#12748=ORIENTED_EDGE ( 'NONE', *, *, #13487, .F. ) ;
#12753=ORIENTED_EDGE ( 'NONE', *, *, #10699, .F. ) ;
#12762=DIRECTION ( 'NONE',  ( -1.000000000000000000, 0.000000000000000000, 0.000000000000000000 ) ) ;
#12771=CARTESIAN_POINT ( 'NONE',  ( 32.07879498588598466, 95.77069236132479091, 15.33800373393474459 ) ) ;
#12776=DIRECTION ( 'NONE',  ( -0.000000000000000000, -0.000000000000000000, 1.000000000000000000 ) ) ;
#12782=DIRECTION ( 'NONE',  ( -1.000000000000000000, 6.308085367188385311E-16, 0.000000000000000000 ) ) ;
#12789=CARTESIAN_POINT ( 'NONE',  ( -30.00000000000000711, 97.48846085563154418, -31.00000000000000000 ) ) ;
#12801=EDGE_CURVE ( 'NONE', #5898, #6159, #4473, .T. ) ;
#12827=VERTEX_POINT ( 'NONE', #4059 ) ;
#12828=DIRECTION ( 'NONE',  ( 0.000000000000000000, 0.000000000000000000, 1.000000000000000000 ) ) ;
#12832=ORIENTED_EDGE ( 'NONE', *, *, #3139, .T. ) ;
#12836=CARTESIAN_POINT ( 'NONE',  ( 25.00000000000000000, 81.24038404635960831, -16.00000000000000000 ) ) ;
#12838=CARTESIAN_POINT ( 'NONE',  ( -7.830013896347489677, 106.7136370351865935, 19.99999999999999289 ) ) ;
#12839=FACE_OUTER_BOUND ( 'NONE', #6827, .T. ) ;
#12843=LINE ( 'NONE', #14061, #10227 ) ;
#12844=ORIENTED_EDGE ( 'NONE', *, *, #1854, .T. ) ;
#12845=ADVANCED_FACE ( 'NONE', ( #5631 ), #10616, .F. ) ;
#12850=AXIS2_PLACEMENT_3D ( 'NONE', #9547, #216, #6345 ) ;
#12880=CYLINDRICAL_SURFACE ( 'NONE', #10014, 95.00000000000001421 ) ;
#12883=ADVANCED_FACE ( 'NONE', ( #7830 ), #10268, .F. ) ;
#12892=ADVANCED_FACE ( 'NONE', ( #7910 ), #13606, .F. ) ;
#12893=EDGE_CURVE ( 'NONE', #5584, #10382, #4716, .T. ) ;
#12894=AXIS2_PLACEMENT_3D ( 'NONE', #11122, #717, #7148 ) ;
#12897=VERTEX_POINT ( 'NONE', #2072 ) ;
#12898=DIRECTION ( 'NONE',  ( 0.9557692240748186796, -0.2941176470588243719, 0.000000000000000000 ) ) ;
#12900=AXIS2_PLACEMENT_3D ( 'NONE', #5775, #4577, #3590 ) ;
#12903=EDGE_CURVE ( 'NONE', #8404, #1158, #10674, .T. ) ;
#12907=EDGE_LOOP ( 'NONE', ( #1040, #10835, #2286, #12635 ) ) ;
#12911=ORIENTED_EDGE ( 'NONE', *, *, #12903, .F. ) ;
#12926=CARTESIAN_POINT ( 'NONE',  ( -12.33230428938080259, 106.2869539367523544, -16.29453878845857062 ) ) ;
#12928=CIRCLE ( 'NONE', #4450, 102.0000000000000142 ) ;
#12929=CARTESIAN_POINT ( 'NONE',  ( 5.204748896376250896E-15, 85.00000000000000000, 46.00000000000000000 ) ) ;
#12934=DIRECTION ( 'NONE',  ( -1.000000000000000000, 0.000000000000000000, 0.000000000000000000 ) ) ;
#12936=ADVANCED_FACE ( 'NONE', ( #3213, #942 ), #10186, .T. ) ;
#12947=ADVANCED_FACE ( 'NONE', ( #298 ), #1437, .F. ) ;
#12952=ORIENTED_EDGE ( 'NONE', *, *, #1125, .F. ) ;
#12955=CARTESIAN_POINT ( 'NONE',  ( 10.55213320575002101, 106.4787665061024597, 18.97395805252363843 ) ) ;
#12956=DIRECTION ( 'NONE',  ( 1.000000000000000000, 0.000000000000000000, 0.000000000000000000 ) ) ;
#12960=DIRECTION ( 'NONE',  ( 0.000000000000000000, 0.000000000000000000, -1.000000000000000000 ) ) ;
#12961=TOROIDAL_SURFACE ( 'NONE', #11274, 17.00000000000000000, 5.000000000000000000 ) ;
#12980=CIRCLE ( 'NONE', #14428, 22.00000000000001421 ) ;
#12981=CARTESIAN_POINT ( 'NONE',  ( -12.05075418994416125, 74.02560756970278533, -17.09116503294089640 ) ) ;
#12982=DIRECTION ( 'NONE',  ( -0.000000000000000000, -0.000000000000000000, 1.000000000000000000 ) ) ;
#12992=DIRECTION ( 'NONE',  ( -1.000000000000000000, 0.000000000000000000, 0.000000000000000000 ) ) ;
#12993=CIRCLE ( 'NONE', #6916, 5.000000000000001776 ) ;
#12997=CARTESIAN_POINT ( 'NONE',  ( 32.45028783375101966, 101.9412720646926118, -14.06019896931748647 ) ) ;
#13025=DIRECTION ( 'NONE',  ( 0.000000000000000000, -1.000000000000000000, -0.000000000000000000 ) ) ;
#13026=EDGE_CURVE ( 'NONE', #1392, #6713, #13053, .T. ) ;
#13031=ORIENTED_EDGE ( 'NONE', *, *, #10929, .F. ) ;
#13032=CARTESIAN_POINT ( 'NONE',  ( 5.204748896376250896E-15, 85.00000000000000000, 31.00000000000000000 ) ) ;
#13036=CARTESIAN_POINT ( 'NONE',  ( -31.56034153936678521, 95.94279256428042402, -14.97248702055886582 ) ) ;
#13043=EDGE_CURVE ( 'NONE', #5260, #3630, #599, .T. ) ;
#13046=ORIENTED_EDGE ( 'NONE', *, *, #2359, .T. ) ;
#13053=LINE ( 'NONE', #8634, #9233 ) ;
#13080=CARTESIAN_POINT ( 'NONE',  ( 31.47058823529413729, 102.2673069760056563, 10.99999999999999645 ) ) ;
#13081=EDGE_CURVE ( 'NONE', #6653, #8389, #8502, .T. ) ;
#13088=DIRECTION ( 'NONE',  ( 0.2941176470588238168, -0.9557692240748187906, 0.000000000000000000 ) ) ;
#13089=AXIS2_PLACEMENT_3D ( 'NONE', #7424, #7343, #1513 ) ;
#13096=AXIS2_PLACEMENT_3D ( 'NONE', #833, #6430, #6496 ) ;
#13097=CARTESIAN_POINT ( 'NONE',  ( -12.39897948556635754, 100.2360479454198696, 16.00000000000000000 ) ) ;
#13103=CYLINDRICAL_SURFACE ( 'NONE', #13699, 5.000000000000000888 ) ;
#13108=CARTESIAN_POINT ( 'NONE',  ( -29.70588235294118107, 96.53269163155674448, -11.33021710499463630 ) ) ;
#13132=DIRECTION ( 'NONE',  ( -0.000000000000000000, -0.000000000000000000, -1.000000000000000000 ) ) ;
#13139=CARTESIAN_POINT ( 'NONE',  ( 0.000000000000000000, 0.000000000000000000, 23.50000000000000355 ) ) ;
#13150=CIRCLE ( 'NONE', #8012, 75.00000000000001421 ) ;
#13153=CARTESIAN_POINT ( 'NONE',  ( -11.47554877443044141, 106.3830115231064184, -18.04988257186027667 ) ) ;
#13156=DIRECTION ( 'NONE',  ( -1.000000000000000000, 0.000000000000000000, -0.000000000000000000 ) ) ;
#13158=ORIENTED_EDGE ( 'NONE', *, *, #13546, .T. ) ;
#13164=CARTESIAN_POINT ( 'NONE',  ( -33.32958405265415536, 101.6044047647130384, -14.99207720203048844 ) ) ;
#13179=ADVANCED_FACE ( 'NONE', ( #11308 ), #910, .F. ) ;
#13182=CARTESIAN_POINT ( 'NONE',  ( -42.00000000000000000, 81.24038404635962252, -31.00000000000000000 ) ) ;
#13187=CARTESIAN_POINT ( 'NONE',  ( -34.44830544488820578, 94.94374256356073261, -16.00000000000000000 ) ) ;
#13189=EDGE_CURVE ( 'NONE', #14956, #11572, #1638, .T. ) ;
#13190=AXIS2_PLACEMENT_3D ( 'NONE', #2017, #8847, #1870 ) ;
#13197=DIRECTION ( 'NONE',  ( -1.000000000000000000, -1.332267629550187849E-14, 0.000000000000000000 ) ) ;
#13200=TOROIDAL_SURFACE ( 'NONE', #13935, 102.0000000000000142, 5.000000000000000000 ) ;
#13204=DIRECTION ( 'NONE',  ( 0.000000000000000000, 0.000000000000000000, 1.000000000000000000 ) ) ;
#13208=DIRECTION ( 'NONE',  ( -1.000000000000000000, 0.000000000000000000, 0.000000000000000000 ) ) ;
#13212=CIRCLE ( 'NONE', #6644, 22.00000000000001421 ) ;
#13214=ORIENTED_EDGE ( 'NONE', *, *, #5698, .F. ) ;
#13215=AXIS2_PLACEMENT_3D ( 'NONE', #7107, #293, #9842 ) ;
#13216=ORIENTED_EDGE ( 'NONE', *, *, #3078, .T. ) ;
#13237=CARTESIAN_POINT ( 'NONE',  ( -4.999999999999996447, 85.00000000000000000, 46.00000000000000000 ) ) ;
#13240=ORIENTED_EDGE ( 'NONE', *, *, #2918, .F. ) ;
#13246=VERTEX_POINT ( 'NONE', #2698 ) ;
#13248=CARTESIAN_POINT ( 'NONE',  ( 12.39897948556635754, 100.2360479454198696, 16.00000000000000000 ) ) ;
#13255=ORIENTED_EDGE ( 'NONE', *, *, #7630, .T. ) ;
#13284=CARTESIAN_POINT ( 'NONE',  ( 36.08010649850015739, 100.2464683348682541, -16.00000000000000000 ) ) ;
#13289=VERTEX_POINT ( 'NONE', #9657 ) ;
#13331=EDGE_CURVE ( 'NONE', #14691, #5358, #7695, .T. ) ;
#13338=ORIENTED_EDGE ( 'NONE', *, *, #382, .F. ) ;
#13344=DIRECTION ( 'NONE',  ( 1.000000000000000000, 0.000000000000000000, 0.000000000000000000 ) ) ;
#13369=PRODUCT_DEFINITION_SHAPE ( 'NONE', 'NONE',  #8937 ) ;
#13375=CARTESIAN_POINT ( 'NONE',  ( 29.95202887341198661, 96.45668229681564299, -12.61733007774791560 ) ) ;
#13380=CARTESIAN_POINT ( 'NONE',  ( 11.26445476358325237, 106.4056658731563942, 18.30680964731275040 ) ) ;
#13387=CARTESIAN_POINT ( 'NONE',  ( -11.63111172283970518, 94.28541358805125583, 17.83102282485376833 ) ) ;
#13390=CARTESIAN_POINT ( 'NONE',  ( 11.47770164139309124, 74.11716252799973859, -18.08381726540839196 ) ) ;
#13396=EDGE_CURVE ( 'NONE', #5665, #1495, #11430, .T. ) ;
#13403=DIRECTION ( 'NONE',  ( -1.000000000000000000, 0.000000000000000000, 0.000000000000000000 ) ) ;
#13406=VERTEX_POINT ( 'NONE', #7920 ) ;
#13407=ORIENTED_EDGE ( 'NONE', *, *, #7773, .T. ) ;
#13412=EDGE_CURVE ( 'NONE', #3540, #15011, #803, .T. ) ;
#13426=CARTESIAN_POINT ( 'NONE',  ( -31.47058823529412663, 102.2673069760056421, 11.00000000000000000 ) ) ;
#13430=VERTEX_POINT ( 'NONE', #3080 ) ;
#13432=CARTESIAN_POINT ( 'NONE',  ( -30.19044911324211000, 96.38232397946877938, 13.21859331841449858 ) ) ;
#13441=EDGE_CURVE ( 'NONE', #13246, #14727, #3924, .T. ) ;
#13452=ORIENTED_EDGE ( 'NONE', *, *, #686, .F. ) ;
#13461=DIRECTION ( 'NONE',  ( 1.000000000000000000, 0.000000000000000000, 0.000000000000000000 ) ) ;
#13463=LINE ( 'NONE', #6608, #4592 ) ;
#13469=CARTESIAN_POINT ( 'NONE',  ( 0.000000000000000000, 0.000000000000000000, -23.50000000000000000 ) ) ;
#13475=ORIENTED_EDGE ( 'NONE', *, *, #921, .T. ) ;
#13486=CARTESIAN_POINT ( 'NONE',  ( 8.075974454121990220, 94.65787058575050139, 19.99999999999999289 ) ) ;
#13487=EDGE_CURVE ( 'NONE', #5269, #2264, #9358, .T. ) ;
#13500=CARTESIAN_POINT ( 'NONE',  ( -31.47058823529411953, 102.2673069760056421, 11.33189534135684973 ) ) ;
#13512=EDGE_LOOP ( 'NONE', ( #8267, #5738, #7095, #7628, #9001, #14863, #2498, #4746 ) ) ;
#13514=VERTEX_POINT ( 'NONE', #5940 ) ;
#13533=PRESENTATION_STYLE_ASSIGNMENT (( #7757 ) ) ;
#13536=CARTESIAN_POINT ( 'NONE',  ( 12.26039456458906152, 94.20559340471635323, -16.55589812076405209 ) ) ;
#13542=CARTESIAN_POINT ( 'NONE',  ( 12.39897948556635754, 61.76783392443436327, 16.00000000000000000 ) ) ;
#13546=EDGE_CURVE ( 'NONE', #3127, #14249, #3436, .T. ) ;
#13547=CARTESIAN_POINT ( 'NONE',  ( 10.80089892394231832, 106.4537193389066374, -18.76964747820620261 ) ) ;
#13553=DIRECTION ( 'NONE',  ( -0.000000000000000000, -0.000000000000000000, 1.000000000000000000 ) ) ;
#13556=ORIENTED_EDGE ( 'NONE', *, *, #7306, .F. ) ;
#13558=EDGE_LOOP ( 'NONE', ( #14741, #4419, #10204, #4808 ) ) ;
#13560=CARTESIAN_POINT ( 'NONE',  ( -12.50000000000000000, 100.2235002382176248, 15.33678752976415716 ) ) ;
#13563=DIRECTION ( 'NONE',  ( -0.000000000000000000, -0.000000000000000000, 1.000000000000000000 ) ) ;
#13566=CARTESIAN_POINT ( 'NONE',  ( -31.95756590787640050, 102.1116157579503323, 13.22695225398607732 ) ) ;
#13579=DIRECTION ( 'NONE',  ( -1.000000000000000000, 0.000000000000000000, 0.000000000000000000 ) ) ;
#13601=CARTESIAN_POINT ( 'NONE',  ( -8.635722793752535154, 94.60824746434937538, -19.90313979694426649 ) ) ;
#13606=CYLINDRICAL_SURFACE ( 'NONE', #11263, 5.000000000000000888 ) ;
#13611=DIRECTION ( 'NONE',  ( 1.000000000000000000, 0.000000000000000000, 0.000000000000000000 ) ) ;
#13612=AXIS2_PLACEMENT_3D ( 'NONE', #5863, #8295, #12934 ) ;
#13625=CARTESIAN_POINT ( 'NONE',  ( 8.632958377326435340, 106.6512898904676092, -19.87266383408973525 ) ) ;
#13627=AXIS2_PLACEMENT_3D ( 'NONE', #3338, #4629, #5828 ) ;
#13666=B_SPLINE_CURVE_WITH_KNOTS ( 'NONE', 3,
 ( #11948, #11863, #9350, #3892, #12926, #2440, #8366, #8506, #397, #13153, #5030, #5856, #10493, #92, #323, #3667, #13998, #14141, #6075, #8210 ),
 .UNSPECIFIED., .F., .F.,
 ( 4, 2, 2, 2, 2, 2, 2, 2, 2, 4 ),
 ( 0.000000000000000000, 0.0009783709435495487137, 0.001467556415324328166, 0.001956741887099107836, 0.002935112830648676282, 0.003913483774198245162, 0.004891854717747813608, 0.005870225661297382054, 0.006848596604846951368, 0.007826967548396519814 ),
 .UNSPECIFIED. ) ;
#13674=DIRECTION ( 'NONE',  ( 1.000000000000000000, 0.000000000000000000, 0.000000000000000000 ) ) ;
#13680=CARTESIAN_POINT ( 'NONE',  ( 34.13789039812933623, 95.05637002121841306, 16.00000000000000711 ) ) ;
#13685=TOROIDAL_SURFACE ( 'NONE', #4003, 17.00000000000001066, 5.000000000000000000 ) ;
#13687=VECTOR ( 'NONE', #8923, 1000.000000000000000 ) ;
#13689=DIRECTION ( 'NONE',  ( -1.000000000000000000, 0.000000000000000000, 0.000000000000000000 ) ) ;
#13696=CARTESIAN_POINT ( 'NONE',  ( 9.449524216731116866, 94.52924706620449058, -19.61300924954587188 ) ) ;
#13699=AXIS2_PLACEMENT_3D ( 'NONE', #10971, #6396, #4987 ) ;
#13711=DIRECTION ( 'NONE',  ( -1.000000000000000000, 0.000000000000000000, 0.000000000000000000 ) ) ;
#13714=VECTOR ( 'NONE', #5343, 1000.000000000000000 ) ;
#13720=CARTESIAN_POINT ( 'NONE',  ( 31.47058823529413729, 102.2673069760056563, 10.99999999999999645 ) ) ;
#13721=DIRECTION ( 'NONE',  ( -0.2941176470588243164, -0.9557692240748185686, -0.000000000000000000 ) ) ;
#13722=AXIS2_PLACEMENT_3D ( 'NONE', #9828, #12960, #2707 ) ;
#13724=ADVANCED_FACE ( 'NONE', ( #2275 ), #12130, .F. ) ;
#13731=CARTESIAN_POINT ( 'NONE',  ( -7.500000000000000888, 106.2673515243510991, 20.00000000000000000 ) ) ;
#13732=( LENGTH_UNIT ( ) NAMED_UNIT ( * ) SI_UNIT ( .MILLI., .METRE. ) );
#13733=CARTESIAN_POINT ( 'NONE',  ( -22.05882352941176450, 71.68269180561142662, -23.50000000000000000 ) ) ;
#13757=ORIENTED_EDGE ( 'NONE', *, *, #4157, .T. ) ;
#13758=CARTESIAN_POINT ( 'NONE',  ( 25.00000000000000000, 81.24038404635960831, -16.00000000000000000 ) ) ;
#13785=EDGE_CURVE ( 'NONE', #143, #10570, #2592, .T. ) ;
#13791=ORIENTED_EDGE ( 'NONE', *, *, #2481, .T. ) ;
#13797=VERTEX_POINT ( 'NONE', #6042 ) ;
#13799=CARTESIAN_POINT ( 'NONE',  ( 10.20278626552728873, 74.30320229487229255, 19.21617406370430103 ) ) ;
#13800=CARTESIAN_POINT ( 'NONE',  ( 0.000000000000000000, 0.000000000000000000, 13.50000000000000533 ) ) ;
#13806=EDGE_LOOP ( 'NONE', ( #370, #2108, #9949, #366, #11220, #11930, #4863, #4061, #8330, #5747, #6058 ) ) ;
#13807=CARTESIAN_POINT ( 'NONE',  ( 0.000000000000000000, 0.000000000000000000, 16.00000000000000000 ) ) ;
#13814=ORIENTED_EDGE ( 'NONE', *, *, #10237, .T. ) ;
#13826=AXIS2_PLACEMENT_3D ( 'NONE', #8958, #14903, #7744 ) ;
#13828=VECTOR ( 'NONE', #14008, 1000.000000000000000 ) ;
#13835=CARTESIAN_POINT ( 'NONE',  ( 29.82779671029265245, 96.49509599019864936, 12.13403317654897329 ) ) ;
#13836=CARTESIAN_POINT ( 'NONE',  ( -8.633615064400526506, 62.40799623593410672, 19.90332611805893137 ) ) ;
#13843=DIRECTION ( 'NONE',  ( -0.000000000000000000, -0.000000000000000000, 1.000000000000000000 ) ) ;
#13846=CARTESIAN_POINT ( 'NONE',  ( 5.204748896376250896E-15, 85.00000000000000000, 46.00000000000000000 ) ) ;
#13852=DIRECTION ( 'NONE',  ( -0.2941176470588241498, -0.9557692240748186796, 0.000000000000000000 ) ) ;
#13853=AXIS2_PLACEMENT_3D ( 'NONE', #8766, #1792, #13403 ) ;
#13858=EDGE_LOOP ( 'NONE', ( #6772, #14872, #11387, #5679 ) ) ;
#13866=ORIENTED_EDGE ( 'NONE', *, *, #8427, .F. ) ;
#13869=CARTESIAN_POINT ( 'NONE',  ( -12.07479981346993902, 61.83277384271320187, -17.09860361742227397 ) ) ;
#13880=CARTESIAN_POINT ( 'NONE',  ( 10.88080562889580705, 74.20685544768620900, 18.69467976711750978 ) ) ;
#13891=DIRECTION ( 'NONE',  ( 0.000000000000000000, 0.000000000000000000, -1.000000000000000000 ) ) ;
#13905=VERTEX_POINT ( 'NONE', #4146 ) ;
#13907=ORIENTED_EDGE ( 'NONE', *, *, #506, .T. ) ;
#13914=EDGE_CURVE ( 'NONE', #12897, #11572, #8763, .T. ) ;
#13916=CARTESIAN_POINT ( 'NONE',  ( 31.56034153936680653, 95.94279256428042402, 14.97248702055886582 ) ) ;
#13921=CARTESIAN_POINT ( 'NONE',  ( -11.99124924651179924, 106.3260354126052079, 17.22144562113021138 ) ) ;
#13935=AXIS2_PLACEMENT_3D ( 'NONE', #10107, #5406, #12317 ) ;
#13945=ORIENTED_EDGE ( 'NONE', *, *, #6638, .F. ) ;
#13951=EDGE_LOOP ( 'NONE', ( #5201, #13255, #1784, #13907, #4249 ) ) ;
#13953=AXIS2_PLACEMENT_3D ( 'NONE', #878, #950, #2002 ) ;
#13965=DIRECTION ( 'NONE',  ( 1.000000000000000000, -1.243449787580175325E-14, 0.000000000000000000 ) ) ;
#13974=CARTESIAN_POINT ( 'NONE',  ( -31.47058823529412663, 102.2673069760056421, 25.99999999999999645 ) ) ;
#13976=TOROIDAL_SURFACE ( 'NONE', #2073, 68.00000000000000000, 5.000000000000000000 ) ;
#13977=CARTESIAN_POINT ( 'NONE',  ( -7.499999999999996447, 85.00000000000000000, 46.00000000000000000 ) ) ;
#13981=CARTESIAN_POINT ( 'NONE',  ( 34.48472847331528612, 95.06210339626261430, -10.99999999999999645 ) ) ;
#13983=VERTEX_POINT ( 'NONE', #10126 ) ;
#13985=ORIENTED_EDGE ( 'NONE', *, *, #4157, .F. ) ;
#13988=CARTESIAN_POINT ( 'NONE',  ( 29.86558579037015804, 96.48341332593348341, 12.29240575635729193 ) ) ;
#13992=PLANE ( 'NONE',  #9209 ) ;
#13998=CARTESIAN_POINT ( 'NONE',  ( -8.801203450618842794, 106.6379082728991676, -19.83890680725670919 ) ) ;
#14007=EDGE_LOOP ( 'NONE', ( #10642, #6878, #10876, #761, #15027, #3318 ) ) ;
#14008=DIRECTION ( 'NONE',  ( 0.000000000000000000, -1.000000000000000000, 0.000000000000000000 ) ) ;
#14016=DIRECTION ( 'NONE',  ( -0.000000000000000000, -0.000000000000000000, 1.000000000000000000 ) ) ;
#14027=CARTESIAN_POINT ( 'NONE',  ( -8.636355552181207429, 94.60704768011227372, 19.87755835258713333 ) ) ;
#14040=DIRECTION ( 'NONE',  ( -1.000000000000000000, -1.953992523340275511E-14, 0.000000000000000000 ) ) ;
#14049=DIRECTION ( 'NONE',  ( -0.000000000000000000, -0.000000000000000000, 1.000000000000000000 ) ) ;
#14056=CYLINDRICAL_SURFACE ( 'NONE', #863, 7.500000000000001776 ) ;
#14058=CARTESIAN_POINT ( 'NONE',  ( 7.500000000000000000, 62.55197838597913318, 20.00000000000000000 ) ) ;
#14061=CARTESIAN_POINT ( 'NONE',  ( 12.50000000000000000, 106.2673515243510991, 15.00000000000000000 ) ) ;
#14069=EDGE_LOOP ( 'NONE', ( #10658, #9952, #2367, #4405, #9685, #12844, #1764, #13945 ) ) ;
#14072=( GEOMETRIC_REPRESENTATION_CONTEXT ( 3 ) GLOBAL_UNCERTAINTY_ASSIGNED_CONTEXT ( ( #6389 ) ) GLOBAL_UNIT_ASSIGNED_CONTEXT ( ( #675, #3026, #7713 ) ) REPRESENTATION_CONTEXT ( 'NONE', 'WORKASPACE' ) );
#14079=CARTESIAN_POINT ( 'NONE',  ( -12.50000000000000000, 106.2673515243510991, 15.00000000000000000 ) ) ;
#14083=CYLINDRICAL_SURFACE ( 'NONE', #304, 22.00000000000001421 ) ;
#14085=VERTEX_POINT ( 'NONE', #5866 ) ;
#14091=CARTESIAN_POINT ( 'NONE',  ( 12.33230428938079903, 106.2869539367523402, 16.29453878845856707 ) ) ;
#14104=DIRECTION ( 'NONE',  ( 0.000000000000000000, 0.000000000000000000, 1.000000000000000000 ) ) ;
#14105=VERTEX_POINT ( 'NONE', #179 ) ;
#14116=CARTESIAN_POINT ( 'NONE',  ( -11.45967689402250755, 74.11957758926655515, -18.06636219913714214 ) ) ;
#14123=AXIS2_PLACEMENT_3D ( 'NONE', #7161, #9653, #7459 ) ;
#14138=ADVANCED_FACE ( 'NONE', ( #5186 ), #14371, .F. ) ;
#14141=CARTESIAN_POINT ( 'NONE',  ( -8.156204789939931032, 106.6891793314719905, -19.96764982490488549 ) ) ;
#14142=DIRECTION ( 'NONE',  ( -1.000000000000000000, 0.000000000000000000, 0.000000000000000000 ) ) ;
#14153=CARTESIAN_POINT ( 'NONE',  ( -25.00000000000000000, 81.24038404635962252, 16.00000000000000000 ) ) ;
#14155=EDGE_CURVE ( 'NONE', #14934, #14546, #7449, .T. ) ;
#14163=ORIENTED_EDGE ( 'NONE', *, *, #10202, .F. ) ;
#14166=CYLINDRICAL_SURFACE ( 'NONE', #6079, 22.00000000000000355 ) ;
#14168=LINE ( 'NONE', #4992, #4995 ) ;
#14171=CIRCLE ( 'NONE', #13215, 10.00000000000000178 ) ;
#14173=EDGE_LOOP ( 'NONE', ( #4856, #9097, #5908, #4092 ) ) ;
#14177=CARTESIAN_POINT ( 'NONE',  ( 35.00000000000000000, 81.24038404635960831, -23.50000000000000000 ) ) ;
#14194=CIRCLE ( 'NONE', #7394, 63.00000000000000000 ) ;
#14203=VERTEX_POINT ( 'NONE', #6231 ) ;
#14208=ORIENTED_EDGE ( 'NONE', *, *, #7723, .T. ) ;
#14214=CARTESIAN_POINT ( 'NONE',  ( -7.500000000000000888, 62.55197838597913318, 20.00000000000000000 ) ) ;
#14220=DIRECTION ( 'NONE',  ( 0.2941176470588243164, 0.9557692240748185686, 0.000000000000000000 ) ) ;
#14227=DIRECTION ( 'NONE',  ( -0.000000000000000000, 1.000000000000000000, -0.000000000000000000 ) ) ;
#14233=ORIENTED_EDGE ( 'NONE', *, *, #9815, .T. ) ;
#14235=DIRECTION ( 'NONE',  ( -0.000000000000000000, -0.000000000000000000, 1.000000000000000000 ) ) ;
#14237=FACE_OUTER_BOUND ( 'NONE', #2502, .T. ) ;
#14240=EDGE_CURVE ( 'NONE', #13905, #9614, #6299, .T. ) ;
#14242=DIRECTION ( 'NONE',  ( -1.000000000000000000, 0.000000000000000000, 0.000000000000000000 ) ) ;
#14245=CARTESIAN_POINT ( 'NONE',  ( 8.633615064400526506, 62.40799623593409251, -19.90332611805893137 ) ) ;
#14247=CARTESIAN_POINT ( 'NONE',  ( -30.88253268887307712, 96.16299873708393875, -14.30432816676291985 ) ) ;
#14249=VERTEX_POINT ( 'NONE', #9506 ) ;
#14259=DIRECTION ( 'NONE',  ( 0.000000000000000000, 1.000000000000000000, -0.000000000000000000 ) ) ;
#14262=DIRECTION ( 'NONE',  ( -1.000000000000000000, 0.000000000000000000, 0.000000000000000000 ) ) ;
#14264=DIRECTION ( 'NONE',  ( -0.000000000000000000, 1.000000000000000000, 0.000000000000000000 ) ) ;
#14272=CARTESIAN_POINT ( 'NONE',  ( 33.32140965599872118, 101.6077678005751181, -14.98557208302583099 ) ) ;
#14292=ORIENTED_EDGE ( 'NONE', *, *, #11770, .F. ) ;
#14297=CARTESIAN_POINT ( 'NONE',  ( -7.500000000000000888, 94.70348462437907244, 20.00000000000000000 ) ) ;
#14298=CARTESIAN_POINT ( 'NONE',  ( -7.787692492290227975, 94.68070094645281642, 19.99999999999999645 ) ) ;
#14300=CARTESIAN_POINT ( 'NONE',  ( 19.99999999999999645, 64.99230723708768664, -26.00000000000000000 ) ) ;
#14311=CARTESIAN_POINT ( 'NONE',  ( 11.08335940112994855, 62.01770010158974600, -18.49860775790518730 ) ) ;
#14314=CARTESIAN_POINT ( 'NONE',  ( -31.32121808728248524, 96.02101045561126114, -14.76552927760546829 ) ) ;
#14330=VECTOR ( 'NONE', #14491, 1000.000000000000000 ) ;
#14347=CARTESIAN_POINT ( 'NONE',  ( 31.47058823529413374, 102.2673069760056848, -11.33189534135685328 ) ) ;
#14360=VECTOR ( 'NONE', #13088, 1000.000000000000114 ) ;
#14361=ORIENTED_EDGE ( 'NONE', *, *, #1797, .F. ) ;
#14371=CYLINDRICAL_SURFACE ( 'NONE', #9263, 10.00000000000000178 ) ;
#14389=FACE_OUTER_BOUND ( 'NONE', #12672, .T. ) ;
#14390=CARTESIAN_POINT ( 'NONE',  ( -8.075966873893682063, 74.56617093413656505, 19.99999999999999645 ) ) ;
#14391=AXIS2_PLACEMENT_3D ( 'NONE', #10757, #2019, #5516 ) ;
#14404=FACE_OUTER_BOUND ( 'NONE', #527, .T. ) ;
#14411=AXIS2_PLACEMENT_3D ( 'NONE', #6945, #11603, #5801 ) ;
#14423=CARTESIAN_POINT ( 'NONE',  ( 0.000000000000000000, 0.000000000000000000, 26.00000000000000000 ) ) ;
#14428=AXIS2_PLACEMENT_3D ( 'NONE', #3427, #1220, #2 ) ;
#14432=ADVANCED_FACE ( 'NONE', ( #11714 ), #3356, .T. ) ;
#14437=CARTESIAN_POINT ( 'NONE',  ( -31.47058823529412663, 102.2673069760056421, 31.00000000000000000 ) ) ;
#14454=EDGE_CURVE ( 'NONE', #5062, #5947, #14623, .T. ) ;
#14455=DIRECTION ( 'NONE',  ( -1.000000000000000000, 0.000000000000000000, 0.000000000000000000 ) ) ;
#14459=CARTESIAN_POINT ( 'NONE',  ( 12.07490296461409329, 74.02221379130672574, -17.09816637537096895 ) ) ;
#14460=CARTESIAN_POINT ( 'NONE',  ( 7.500000000000000888, 106.2673515243510991, -20.00000000000000000 ) ) ;
#14461=DIRECTION ( 'NONE',  ( -0.000000000000000000, -0.000000000000000000, 1.000000000000000000 ) ) ;
#14462=CIRCLE ( 'NONE', #394, 22.00000000000001421 ) ;
#14471=EDGE_CURVE ( 'NONE', #4010, #4879, #86, .T. ) ;
#14475=CARTESIAN_POINT ( 'NONE',  ( -32.92366211674482912, 95.48362627681295578, -15.74283067514923751 ) ) ;
#14483=ADVANCED_FACE ( 'NONE', ( #12839 ), #10340, .F. ) ;
#14485=CARTESIAN_POINT ( 'NONE',  ( 12.39897948556635399, 61.76783392443435616, -16.00000000000000000 ) ) ;
#14491=DIRECTION ( 'NONE',  ( -0.000000000000000000, -0.000000000000000000, -1.000000000000000000 ) ) ;
#14498=CARTESIAN_POINT ( 'NONE',  ( -7.500000000000000888, 61.74746958378133144, -20.00000000000000000 ) ) ;
#14508=CARTESIAN_POINT ( 'NONE',  ( 0.000000000000000000, 0.000000000000000000, -79.80561291909842225 ) ) ;
#14526=ADVANCED_FACE ( 'NONE', ( #6752 ), #13992, .T. ) ;
#14528=CARTESIAN_POINT ( 'NONE',  ( -12.26039456458906152, 94.20559340471635323, 16.55589812076405565 ) ) ;
#14530=EDGE_CURVE ( 'NONE', #7147, #4198, #11578, .T. ) ;
#14546=VERTEX_POINT ( 'NONE', #5771 ) ;
#14550=FACE_OUTER_BOUND ( 'NONE', #7068, .T. ) ;
#14558=ORIENTED_EDGE ( 'NONE', *, *, #12502, .T. ) ;
#14559=ORIENTED_EDGE ( 'NONE', *, *, #12893, .T. ) ;
#14569=EDGE_CURVE ( 'NONE', #8389, #13406, #2422, .T. ) ;
#14576=AXIS2_PLACEMENT_3D ( 'NONE', #12305, #687, #4100 ) ;
#14583=FACE_OUTER_BOUND ( 'NONE', #5673, .T. ) ;
#14585=VECTOR ( 'NONE', #7943, 1000.000000000000000 ) ;
#14586=PRODUCT_DEFINITION_CONTEXT ( 'detailed design', #11945, 'design' ) ;
#14590=DIRECTION ( 'NONE',  ( -1.000000000000000000, 0.000000000000000000, 0.000000000000000000 ) ) ;
#14617=CARTESIAN_POINT ( 'NONE',  ( 27.94117647058824616, 90.79807628710781842, -16.00000000000000000 ) ) ;
#14623=CIRCLE ( 'NONE', #63, 63.00000000000000000 ) ;
#14635=DIRECTION ( 'NONE',  ( 1.000000000000000000, 0.000000000000000000, 0.000000000000000000 ) ) ;
#14637=VERTEX_POINT ( 'NONE', #14058 ) ;
#14643=CARTESIAN_POINT ( 'NONE',  ( -12.50000000000000000, 59.24038404635959409, -20.00000000000000000 ) ) ;
#14649=VERTEX_POINT ( 'NONE', #9485 ) ;
#14655=CARTESIAN_POINT ( 'NONE',  ( 22.05882352941176094, 71.68269180561141241, -23.50000000000000000 ) ) ;
#14660=CARTESIAN_POINT ( 'NONE',  ( 5.204748896376250896E-15, 85.00000000000000000, 46.00000000000000000 ) ) ;
#14677=DIRECTION ( 'NONE',  ( -1.000000000000000000, 0.000000000000000000, 0.000000000000000000 ) ) ;
#14680=CARTESIAN_POINT ( 'NONE',  ( -12.07377633196514566, 61.83297368684232964, 17.10072941380094846 ) ) ;
#14691=VERTEX_POINT ( 'NONE', #230 ) ;
#14697=VECTOR ( 'NONE', #2259, 1000.000000000000000 ) ;
#14722=DIRECTION ( 'NONE',  ( -1.000000000000000000, 6.308085367188389255E-16, 0.000000000000000000 ) ) ;
#14727=VERTEX_POINT ( 'NONE', #2882 ) ;
#14729=CARTESIAN_POINT ( 'NONE',  ( -34.64620656398767551, 101.0151817716822507, 15.74933755401541902 ) ) ;
#14734=FACE_OUTER_BOUND ( 'NONE', #10945, .T. ) ;
#14740=CARTESIAN_POINT ( 'NONE',  ( 25.00000000000000000, 81.24038404635960831, -26.00000000000000000 ) ) ;
#14741=ORIENTED_EDGE ( 'NONE', *, *, #13189, .F. ) ;
#14743=DIRECTION ( 'NONE',  ( -1.000000000000000000, 0.000000000000000000, 0.000000000000000000 ) ) ;
#14762=CARTESIAN_POINT ( 'NONE',  ( 10.44268084954786069, 94.42456965614839248, -19.05230465901501091 ) ) ;
#14768=DIRECTION ( 'NONE',  ( 0.000000000000000000, 1.000000000000000000, 0.000000000000000000 ) ) ;
#14772=CARTESIAN_POINT ( 'NONE',  ( 8.154413083459850498, 106.6893057894985617, -19.96764870088429689 ) ) ;
#14777=CYLINDRICAL_SURFACE ( 'NONE', #9832, 5.000000000000000888 ) ;
#14781=AXIS2_PLACEMENT_3D ( 'NONE', #9411, #13843, #14910 ) ;
#14797=CARTESIAN_POINT ( 'NONE',  ( -18.52941176470586981, 60.21346111671361001, 31.00000000000000000 ) ) ;
#14827=CARTESIAN_POINT ( 'NONE',  ( -12.07539369549097863, 94.22990561005788379, -17.09692597381455315 ) ) ;
#14831=CARTESIAN_POINT ( 'NONE',  ( 12.50000000000000000, 40.62019202317980415, 31.00000000000000000 ) ) ;
#14835=ORIENTED_EDGE ( 'NONE', *, *, #1702, .F. ) ;
#14843=ORIENTED_EDGE ( 'NONE', *, *, #844, .T. ) ;
#14858=CARTESIAN_POINT ( 'NONE',  ( 34.65532077583679893, 101.0090414146251590, 15.74457401924681932 ) ) ;
#14861=ORIENTED_EDGE ( 'NONE', *, *, #7259, .F. ) ;
#14863=ORIENTED_EDGE ( 'NONE', *, *, #4469, .T. ) ;
#14864=CARTESIAN_POINT ( 'NONE',  ( 12.05075418994416125, 74.02560756970278533, 17.09116503294089995 ) ) ;
#14867=DIRECTION ( 'NONE',  ( 1.000000000000000000, 0.000000000000000000, 0.000000000000000000 ) ) ;
#14872=ORIENTED_EDGE ( 'NONE', *, *, #2922, .T. ) ;
#14873=CARTESIAN_POINT ( 'NONE',  ( 25.00000000000000000, 81.24038404635960831, -16.00000000000000000 ) ) ;
#14874=FACE_OUTER_BOUND ( 'NONE', #13512, .T. ) ;
#14880=EDGE_CURVE ( 'NONE', #13797, #9064, #1941, .T. ) ;
#14894=DIRECTION ( 'NONE',  ( -1.000000000000000000, -3.552713678800500929E-15, 0.000000000000000000 ) ) ;
#14903=DIRECTION ( 'NONE',  ( 0.000000000000000000, 0.000000000000000000, -1.000000000000000000 ) ) ;
#14907=DIRECTION ( 'NONE',  ( 0.2941176470588238168, -0.9557692240748187906, 0.000000000000000000 ) ) ;
#14910=DIRECTION ( 'NONE',  ( 1.000000000000000000, 0.000000000000000000, 0.000000000000000000 ) ) ;
#14911=( NAMED_UNIT ( * ) SI_UNIT ( $, .STERADIAN. ) SOLID_ANGLE_UNIT ( ) );
#14934=VERTEX_POINT ( 'NONE', #2277 ) ;
#14939=VERTEX_POINT ( 'NONE', #5611 ) ;
#14946=CARTESIAN_POINT ( 'NONE',  ( 0.000000000000000000, 0.000000000000000000, 31.00000000000000000 ) ) ;
#14948=VECTOR ( 'NONE', #8002, 1000.000000000000114 ) ;
#14954=LINE ( 'NONE', #14797, #10128 ) ;
#14955=ORIENTED_EDGE ( 'NONE', *, *, #9964, .T. ) ;
#14956=VERTEX_POINT ( 'NONE', #5539 ) ;
#14958=AXIS2_PLACEMENT_3D ( 'NONE', #4274, #6512, #1899 ) ;
#14968=ORIENTED_EDGE ( 'NONE', *, *, #2587, .T. ) ;
#14984=EDGE_CURVE ( 'NONE', #4528, #27, #11667, .T. ) ;
#14987=DIRECTION ( 'NONE',  ( -0.000000000000000000, -0.000000000000000000, 1.000000000000000000 ) ) ;
#15011=VERTEX_POINT ( 'NONE', #1588 ) ;
#15012=CARTESIAN_POINT ( 'NONE',  ( 12.26010588040893978, 73.99122283359872654, 16.55683232866783783 ) ) ;
#15013=DIRECTION ( 'NONE',  ( -0.000000000000000000, -0.000000000000000000, -1.000000000000000000 ) ) ;
#15020=DIRECTION ( 'NONE',  ( -0.9557692240748189016, 0.2941176470588239833, 0.000000000000000000 ) ) ;
#15021=EDGE_CURVE ( 'NONE', #2772, #10943, #5825, .T. ) ;
#15022=EDGE_CURVE ( 'NONE', #4198, #12536, #1231, .T. ) ;
#15027=ORIENTED_EDGE ( 'NONE', *, *, #6655, .F. ) ;
ENDSEC;
END-ISO-10303-21;
